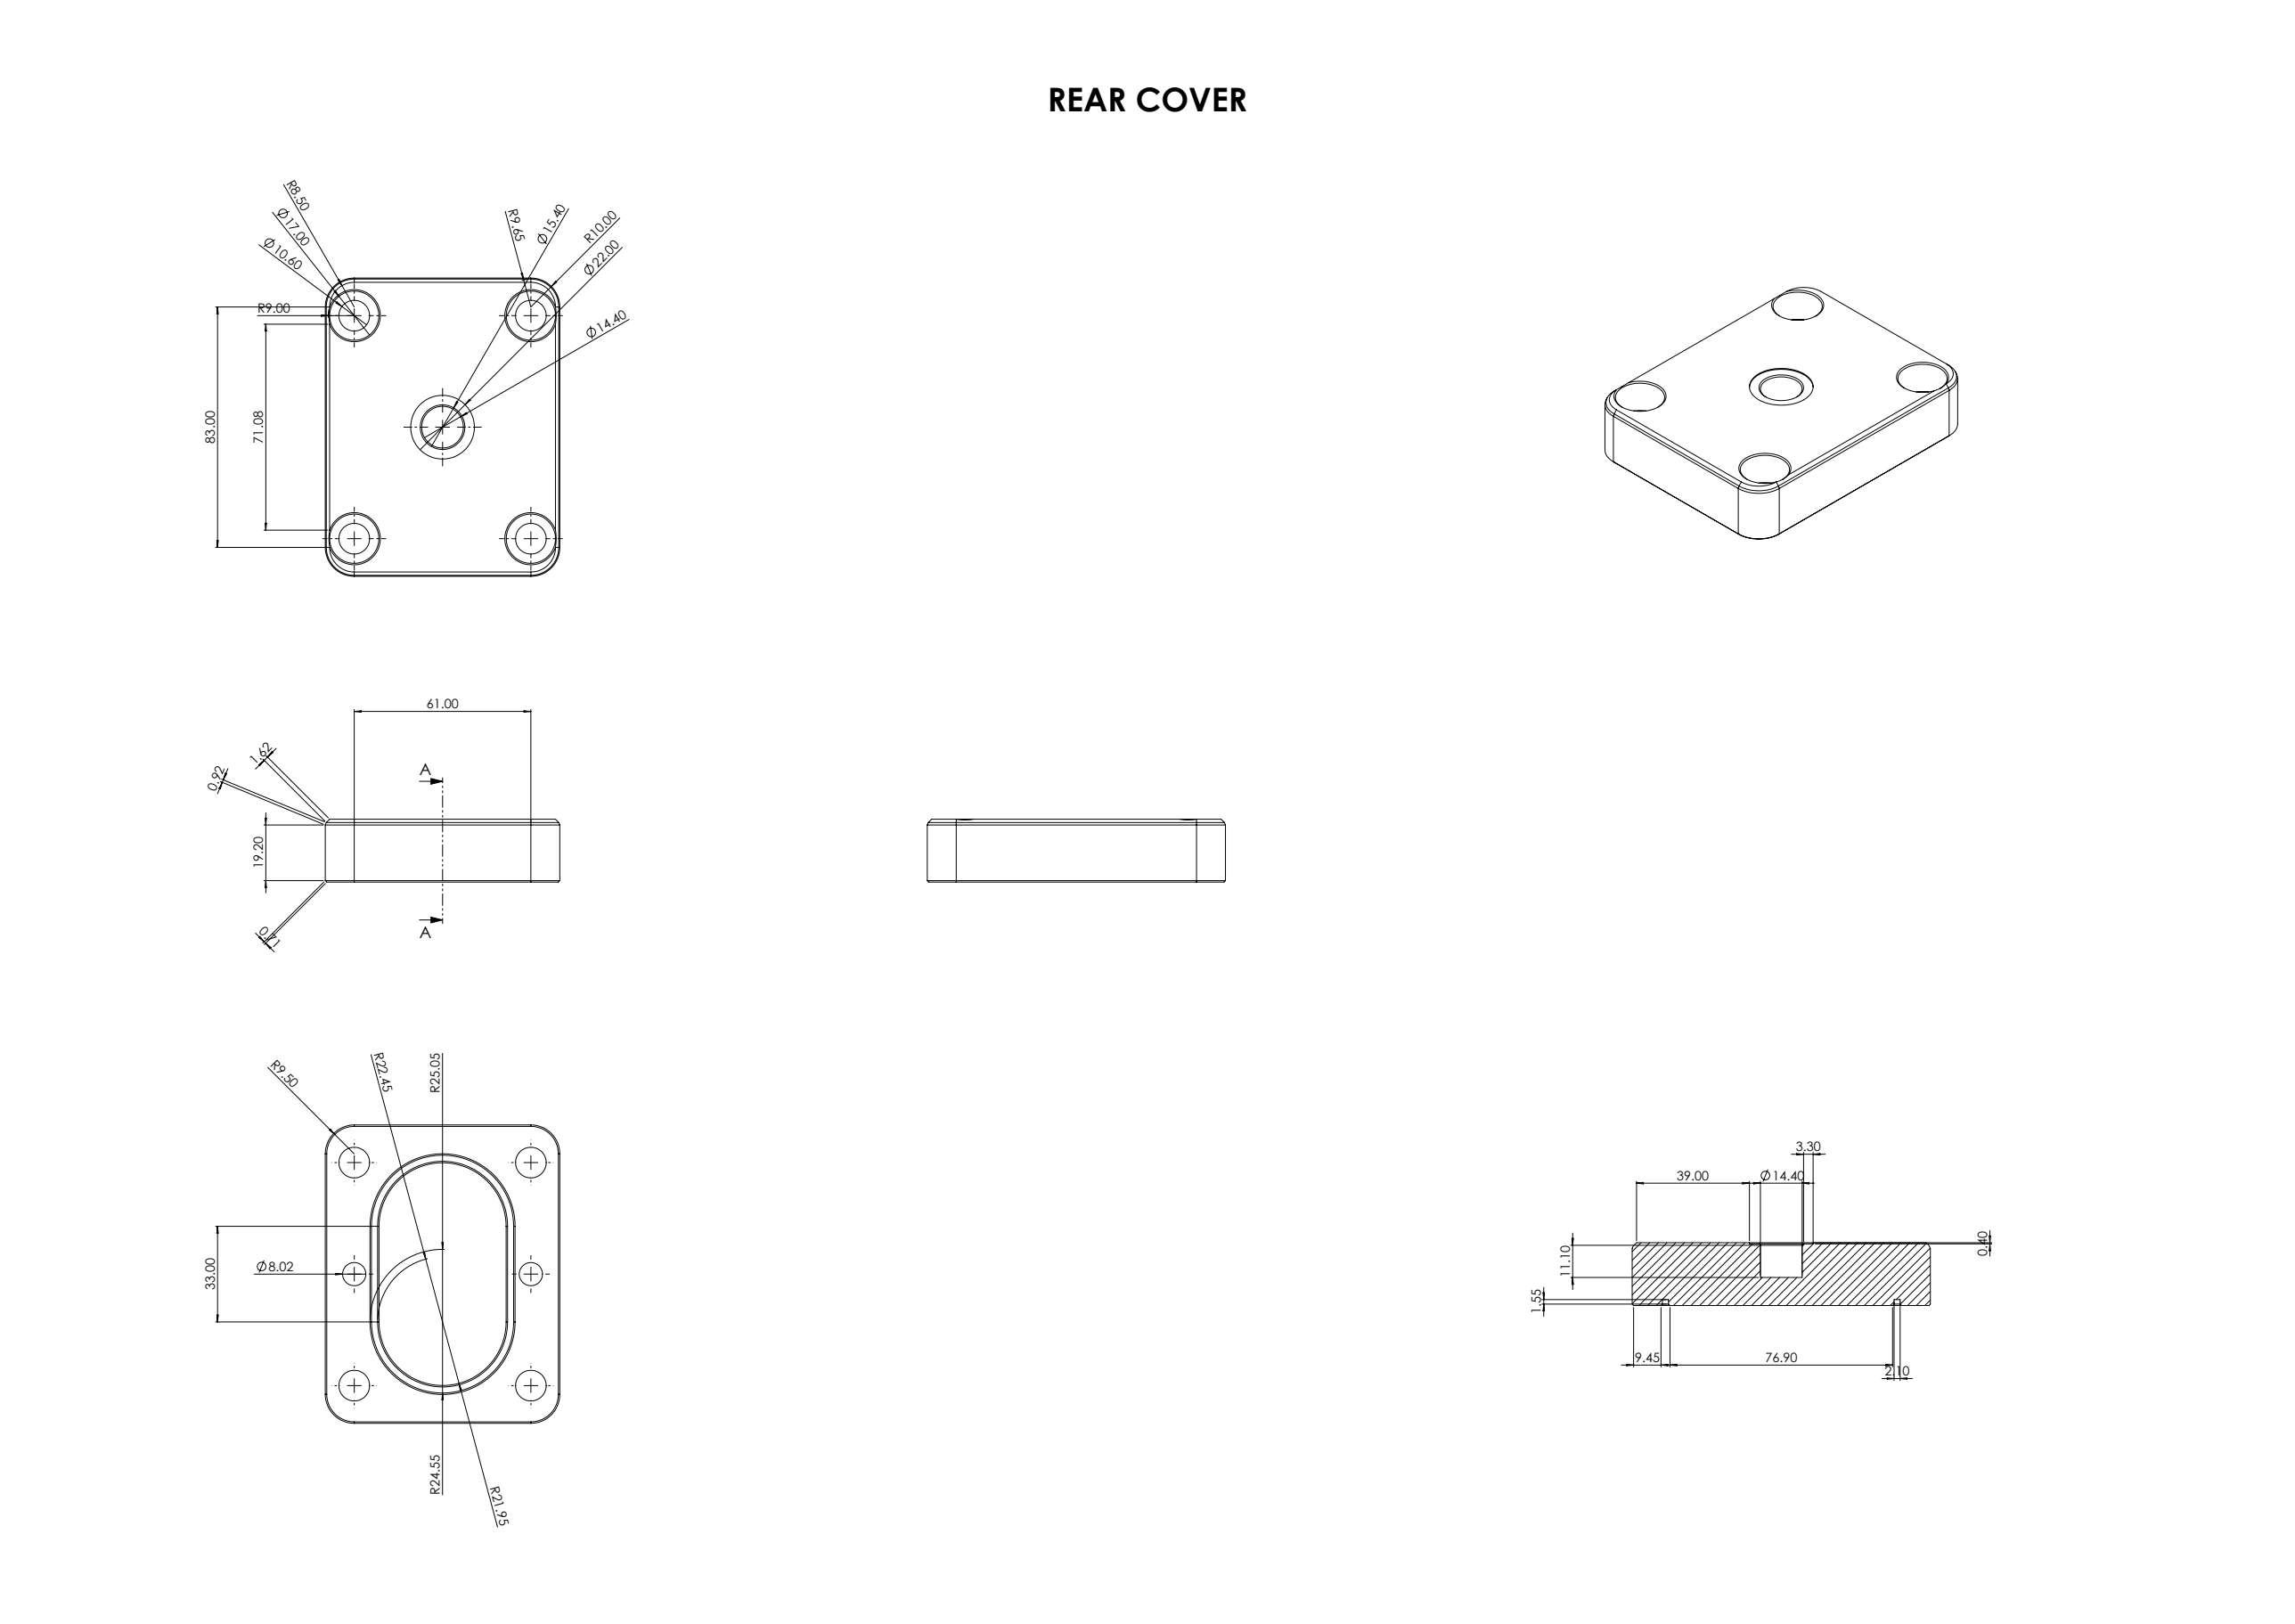
ISO-10303-21;
HEADER;
/* Generated by software containing ST-Developer
 * from STEP Tools, Inc. (www.steptools.com) 
 */

FILE_DESCRIPTION(
/* description */ (''),
/* implementation_level */ '2;1');

FILE_NAME(
/* name */ '03_Rear_Cover.step',
/* time_stamp */ '2026-10-26T06:59:52-07:00',
/* author */ (''),
/* organization */ (''),
/* preprocessor_version */ 'ST-DEVELOPER v20.2',
/* originating_system */ 'Autodesk Translation Framework v15.15.0.0',
/* authorisation */ '');

FILE_SCHEMA (('AUTOMOTIVE_DESIGN { 1 0 10303 214 3 1 1 }'));
ENDSEC;

DATA;
#10=MECHANICAL_DESIGN_GEOMETRIC_PRESENTATION_REPRESENTATION('',(#166),#46395);
#115=(
BOUNDED_CURVE()
B_SPLINE_CURVE(2,(#35773,#35774,#35775),.UNSPECIFIED.,.F.,.F.)
B_SPLINE_CURVE_WITH_KNOTS((3,3),(0.,0.297909382195316),.UNSPECIFIED.)
CURVE()
GEOMETRIC_REPRESENTATION_ITEM()
RATIONAL_B_SPLINE_CURVE((1.,1.,1.))
REPRESENTATION_ITEM('')
);
#116=(
BOUNDED_CURVE()
B_SPLINE_CURVE(2,(#35780,#35781,#35782),.UNSPECIFIED.,.F.,.F.)
B_SPLINE_CURVE_WITH_KNOTS((3,3),(0.297909382195316,0.595818764390632),
 .UNSPECIFIED.)
CURVE()
GEOMETRIC_REPRESENTATION_ITEM()
RATIONAL_B_SPLINE_CURVE((1.,1.,1.))
REPRESENTATION_ITEM('')
);
#117=(
BOUNDED_CURVE()
B_SPLINE_CURVE(2,(#35788,#35789,#35790),.UNSPECIFIED.,.F.,.F.)
B_SPLINE_CURVE_WITH_KNOTS((3,3),(0.297909382195316,0.595818764390632),
 .UNSPECIFIED.)
CURVE()
GEOMETRIC_REPRESENTATION_ITEM()
RATIONAL_B_SPLINE_CURVE((1.,1.,1.))
REPRESENTATION_ITEM('')
);
#118=(
BOUNDED_CURVE()
B_SPLINE_CURVE(2,(#35792,#35793,#35794),.UNSPECIFIED.,.F.,.F.)
B_SPLINE_CURVE_WITH_KNOTS((3,3),(0.,0.297909382195316),.UNSPECIFIED.)
CURVE()
GEOMETRIC_REPRESENTATION_ITEM()
RATIONAL_B_SPLINE_CURVE((1.,1.,1.))
REPRESENTATION_ITEM('')
);
#119=(
BOUNDED_CURVE()
B_SPLINE_CURVE(2,(#35820,#35821,#35822),.UNSPECIFIED.,.F.,.F.)
B_SPLINE_CURVE_WITH_KNOTS((3,3),(0.,0.297909382195316),.UNSPECIFIED.)
CURVE()
GEOMETRIC_REPRESENTATION_ITEM()
RATIONAL_B_SPLINE_CURVE((1.,1.,1.))
REPRESENTATION_ITEM('')
);
#120=(
BOUNDED_CURVE()
B_SPLINE_CURVE(2,(#35829,#35830,#35831),.UNSPECIFIED.,.F.,.F.)
B_SPLINE_CURVE_WITH_KNOTS((3,3),(0.297909382195316,0.595818764390632),
 .UNSPECIFIED.)
CURVE()
GEOMETRIC_REPRESENTATION_ITEM()
RATIONAL_B_SPLINE_CURVE((1.,1.,1.))
REPRESENTATION_ITEM('')
);
#121=(
BOUNDED_CURVE()
B_SPLINE_CURVE(2,(#35837,#35838,#35839),.UNSPECIFIED.,.F.,.F.)
B_SPLINE_CURVE_WITH_KNOTS((3,3),(0.297909382195316,0.595818764390632),
 .UNSPECIFIED.)
CURVE()
GEOMETRIC_REPRESENTATION_ITEM()
RATIONAL_B_SPLINE_CURVE((1.,1.,1.))
REPRESENTATION_ITEM('')
);
#122=(
BOUNDED_CURVE()
B_SPLINE_CURVE(2,(#35841,#35842,#35843),.UNSPECIFIED.,.F.,.F.)
B_SPLINE_CURVE_WITH_KNOTS((3,3),(0.,0.297909382195316),.UNSPECIFIED.)
CURVE()
GEOMETRIC_REPRESENTATION_ITEM()
RATIONAL_B_SPLINE_CURVE((1.,1.,1.))
REPRESENTATION_ITEM('')
);
#138=SHAPE_REPRESENTATION_RELATIONSHIP('SRR','None',#46458,#152);
#152=ADVANCED_BREP_SHAPE_REPRESENTATION('',(#180),#46383);
#166=STYLED_ITEM('',(#46610),#180);
#180=MANIFOLD_SOLID_BREP('Body1',#24939);
#494=CYLINDRICAL_SURFACE('',#25568,7.2);
#495=CYLINDRICAL_SURFACE('',#25578,24.55);
#496=CYLINDRICAL_SURFACE('',#25600,22.45);
#497=CYLINDRICAL_SURFACE('',#25608,8.5);
#498=CYLINDRICAL_SURFACE('',#25613,8.5);
#499=CYLINDRICAL_SURFACE('',#25620,8.5);
#500=CYLINDRICAL_SURFACE('',#25626,8.5);
#501=CYLINDRICAL_SURFACE('',#25641,9.99999999999999);
#502=CYLINDRICAL_SURFACE('',#25644,9.99999999999999);
#503=CYLINDRICAL_SURFACE('',#25672,22.45);
#504=CYLINDRICAL_SURFACE('',#25675,24.55);
#505=CYLINDRICAL_SURFACE('',#25679,11.);
#506=CYLINDRICAL_SURFACE('',#25681,4.01);
#507=CYLINDRICAL_SURFACE('',#25684,4.01);
#508=CYLINDRICAL_SURFACE('',#25687,5.3);
#509=CYLINDRICAL_SURFACE('',#25689,5.3);
#510=CYLINDRICAL_SURFACE('',#25691,5.3);
#511=CYLINDRICAL_SURFACE('',#25693,5.3);
#512=CYLINDRICAL_SURFACE('',#25699,9.99999999999999);
#513=CYLINDRICAL_SURFACE('',#25701,10.);
#631=FACE_BOUND('',#3353,.T.);
#632=FACE_BOUND('',#3362,.T.);
#633=FACE_BOUND('',#3363,.T.);
#634=FACE_BOUND('',#3364,.T.);
#635=FACE_BOUND('',#3365,.T.);
#636=FACE_BOUND('',#3366,.T.);
#637=FACE_BOUND('',#3367,.T.);
#638=FACE_BOUND('',#3368,.T.);
#639=FACE_BOUND('',#3413,.T.);
#640=FACE_BOUND('',#3419,.T.);
#641=FACE_BOUND('',#3431,.T.);
#642=FACE_BOUND('',#3433,.T.);
#643=FACE_BOUND('',#3435,.T.);
#644=FACE_BOUND('',#3437,.T.);
#778=PLANE('',#25566);
#779=PLANE('',#25570);
#780=PLANE('',#25574);
#781=PLANE('',#25580);
#782=PLANE('',#25581);
#783=PLANE('',#25592);
#784=PLANE('',#25596);
#785=PLANE('',#25602);
#786=PLANE('',#25603);
#787=PLANE('',#25607);
#788=PLANE('',#25619);
#789=PLANE('',#25630);
#790=PLANE('',#25633);
#791=PLANE('',#25636);
#792=PLANE('',#25639);
#793=PLANE('',#25640);
#794=PLANE('',#25643);
#795=PLANE('',#25646);
#796=PLANE('',#25649);
#797=PLANE('',#25652);
#798=PLANE('',#25656);
#799=PLANE('',#25662);
#800=PLANE('',#25667);
#801=PLANE('',#25670);
#802=PLANE('',#25674);
#803=PLANE('',#25677);
#804=PLANE('',#25678);
#805=PLANE('',#25680);
#806=PLANE('',#25683);
#807=PLANE('',#25686);
#808=PLANE('',#25695);
#809=PLANE('',#25696);
#810=PLANE('',#25697);
#811=PLANE('',#25698);
#812=PLANE('',#25700);
#813=PLANE('',#25702);
#1975=FACE_OUTER_BOUND('',#3351,.T.);
#1976=FACE_OUTER_BOUND('',#3352,.T.);
#1977=FACE_OUTER_BOUND('',#3354,.T.);
#1978=FACE_OUTER_BOUND('',#3355,.T.);
#1979=FACE_OUTER_BOUND('',#3356,.T.);
#1980=FACE_OUTER_BOUND('',#3357,.T.);
#1981=FACE_OUTER_BOUND('',#3358,.T.);
#1982=FACE_OUTER_BOUND('',#3359,.T.);
#1983=FACE_OUTER_BOUND('',#3360,.T.);
#1984=FACE_OUTER_BOUND('',#3361,.T.);
#1985=FACE_OUTER_BOUND('',#3369,.T.);
#1986=FACE_OUTER_BOUND('',#3370,.T.);
#1987=FACE_OUTER_BOUND('',#3371,.T.);
#1988=FACE_OUTER_BOUND('',#3372,.T.);
#1989=FACE_OUTER_BOUND('',#3373,.T.);
#1990=FACE_OUTER_BOUND('',#3374,.T.);
#1991=FACE_OUTER_BOUND('',#3375,.T.);
#1992=FACE_OUTER_BOUND('',#3376,.T.);
#1993=FACE_OUTER_BOUND('',#3377,.T.);
#1994=FACE_OUTER_BOUND('',#3378,.T.);
#1995=FACE_OUTER_BOUND('',#3379,.T.);
#1996=FACE_OUTER_BOUND('',#3380,.T.);
#1997=FACE_OUTER_BOUND('',#3381,.T.);
#1998=FACE_OUTER_BOUND('',#3382,.T.);
#1999=FACE_OUTER_BOUND('',#3383,.T.);
#2000=FACE_OUTER_BOUND('',#3384,.T.);
#2001=FACE_OUTER_BOUND('',#3385,.T.);
#2002=FACE_OUTER_BOUND('',#3386,.T.);
#2003=FACE_OUTER_BOUND('',#3387,.T.);
#2004=FACE_OUTER_BOUND('',#3388,.T.);
#2005=FACE_OUTER_BOUND('',#3389,.T.);
#2006=FACE_OUTER_BOUND('',#3390,.T.);
#2007=FACE_OUTER_BOUND('',#3391,.T.);
#2008=FACE_OUTER_BOUND('',#3392,.T.);
#2009=FACE_OUTER_BOUND('',#3393,.T.);
#2010=FACE_OUTER_BOUND('',#3394,.T.);
#2011=FACE_OUTER_BOUND('',#3395,.T.);
#2012=FACE_OUTER_BOUND('',#3396,.T.);
#2013=FACE_OUTER_BOUND('',#3397,.T.);
#2014=FACE_OUTER_BOUND('',#3398,.T.);
#2015=FACE_OUTER_BOUND('',#3399,.T.);
#2016=FACE_OUTER_BOUND('',#3400,.T.);
#2017=FACE_OUTER_BOUND('',#3401,.T.);
#2018=FACE_OUTER_BOUND('',#3402,.T.);
#2019=FACE_OUTER_BOUND('',#3403,.T.);
#2020=FACE_OUTER_BOUND('',#3404,.T.);
#2021=FACE_OUTER_BOUND('',#3405,.T.);
#2022=FACE_OUTER_BOUND('',#3406,.T.);
#2023=FACE_OUTER_BOUND('',#3407,.T.);
#2024=FACE_OUTER_BOUND('',#3408,.T.);
#2025=FACE_OUTER_BOUND('',#3409,.T.);
#2026=FACE_OUTER_BOUND('',#3410,.T.);
#2027=FACE_OUTER_BOUND('',#3411,.T.);
#2028=FACE_OUTER_BOUND('',#3412,.T.);
#2029=FACE_OUTER_BOUND('',#3414,.T.);
#2030=FACE_OUTER_BOUND('',#3415,.T.);
#2031=FACE_OUTER_BOUND('',#3416,.T.);
#2032=FACE_OUTER_BOUND('',#3417,.T.);
#2033=FACE_OUTER_BOUND('',#3418,.T.);
#2034=FACE_OUTER_BOUND('',#3420,.T.);
#2035=FACE_OUTER_BOUND('',#3421,.T.);
#2036=FACE_OUTER_BOUND('',#3422,.T.);
#2037=FACE_OUTER_BOUND('',#3423,.T.);
#2038=FACE_OUTER_BOUND('',#3424,.T.);
#2039=FACE_OUTER_BOUND('',#3425,.T.);
#2040=FACE_OUTER_BOUND('',#3426,.T.);
#2041=FACE_OUTER_BOUND('',#3427,.T.);
#2042=FACE_OUTER_BOUND('',#3428,.T.);
#2043=FACE_OUTER_BOUND('',#3429,.T.);
#2044=FACE_OUTER_BOUND('',#3430,.T.);
#2045=FACE_OUTER_BOUND('',#3432,.T.);
#2046=FACE_OUTER_BOUND('',#3434,.T.);
#2047=FACE_OUTER_BOUND('',#3436,.T.);
#2048=FACE_OUTER_BOUND('',#3438,.T.);
#2049=FACE_OUTER_BOUND('',#3439,.T.);
#2050=FACE_OUTER_BOUND('',#3440,.T.);
#2051=FACE_OUTER_BOUND('',#3441,.T.);
#3351=EDGE_LOOP('',(#17582,#17583,#17584,#17585));
#3352=EDGE_LOOP('',(#17586));
#3353=EDGE_LOOP('',(#17587));
#3354=EDGE_LOOP('',(#17588,#17589,#17590,#17591));
#3355=EDGE_LOOP('',(#17592,#17593,#17594,#17595));
#3356=EDGE_LOOP('',(#17596,#17597,#17598,#17599));
#3357=EDGE_LOOP('',(#17600,#17601,#17602,#17603));
#3358=EDGE_LOOP('',(#17604,#17605,#17606,#17607));
#3359=EDGE_LOOP('',(#17608,#17609,#17610,#17611));
#3360=EDGE_LOOP('',(#17612,#17613,#17614,#17615));
#3361=EDGE_LOOP('',(#17616,#17617,#17618,#17619,#17620,#17621,#17622,#17623));
#3362=EDGE_LOOP('',(#17624));
#3363=EDGE_LOOP('',(#17625));
#3364=EDGE_LOOP('',(#17626));
#3365=EDGE_LOOP('',(#17627));
#3366=EDGE_LOOP('',(#17628));
#3367=EDGE_LOOP('',(#17629));
#3368=EDGE_LOOP('',(#17630,#17631,#17632,#17633));
#3369=EDGE_LOOP('',(#17634,#17635,#17636,#17637));
#3370=EDGE_LOOP('',(#17638,#17639,#17640,#17641));
#3371=EDGE_LOOP('',(#17642,#17643,#17644,#17645));
#3372=EDGE_LOOP('',(#17646,#17647,#17648,#17649));
#3373=EDGE_LOOP('',(#17650,#17651,#17652,#17653));
#3374=EDGE_LOOP('',(#17654,#17655,#17656,#17657));
#3375=EDGE_LOOP('',(#17658,#17659,#17660,#17661));
#3376=EDGE_LOOP('',(#17662,#17663,#17664,#17665,#17666,#17667));
#3377=EDGE_LOOP('',(#17668,#17669,#17670,#17671,#17672,#17673,#17674,#17675,
#17676,#17677));
#3378=EDGE_LOOP('',(#17678,#17679,#17680,#17681));
#3379=EDGE_LOOP('',(#17682,#17683,#17684,#17685,#17686,#17687));
#3380=EDGE_LOOP('',(#17688,#17689,#17690,#17691));
#3381=EDGE_LOOP('',(#17692,#17693,#17694,#17695,#17696,#17697,#17698));
#3382=EDGE_LOOP('',(#17699,#17700,#17701,#17702,#17703,#17704,#17705,#17706,
#17707,#17708));
#3383=EDGE_LOOP('',(#17709,#17710,#17711,#17712,#17713));
#3384=EDGE_LOOP('',(#17714,#17715,#17716,#17717,#17718,#17719,#17720));
#3385=EDGE_LOOP('',(#17721,#17722,#17723,#17724,#17725));
#3386=EDGE_LOOP('',(#17726,#17727,#17728,#17729));
#3387=EDGE_LOOP('',(#17730,#17731,#17732,#17733));
#3388=EDGE_LOOP('',(#17734,#17735,#17736,#17737));
#3389=EDGE_LOOP('',(#17738,#17739,#17740,#17741));
#3390=EDGE_LOOP('',(#17742,#17743,#17744,#17745));
#3391=EDGE_LOOP('',(#17746,#17747,#17748,#17749));
#3392=EDGE_LOOP('',(#17750,#17751,#17752,#17753));
#3393=EDGE_LOOP('',(#17754,#17755,#17756,#17757));
#3394=EDGE_LOOP('',(#17758,#17759,#17760,#17761));
#3395=EDGE_LOOP('',(#17762,#17763,#17764,#17765));
#3396=EDGE_LOOP('',(#17766,#17767,#17768,#17769));
#3397=EDGE_LOOP('',(#17770,#17771,#17772,#17773));
#3398=EDGE_LOOP('',(#17774,#17775,#17776,#17777));
#3399=EDGE_LOOP('',(#17778,#17779,#17780,#17781));
#3400=EDGE_LOOP('',(#17782,#17783,#17784,#17785));
#3401=EDGE_LOOP('',(#17786,#17787,#17788,#17789));
#3402=EDGE_LOOP('',(#17790,#17791,#17792,#17793));
#3403=EDGE_LOOP('',(#17794,#17795,#17796,#17797));
#3404=EDGE_LOOP('',(#17798,#17799,#17800,#17801));
#3405=EDGE_LOOP('',(#17802,#17803,#17804,#17805));
#3406=EDGE_LOOP('',(#17806,#17807,#17808,#17809));
#3407=EDGE_LOOP('',(#17810,#17811,#17812,#17813));
#3408=EDGE_LOOP('',(#17814,#17815,#17816,#17817));
#3409=EDGE_LOOP('',(#17818,#17819,#17820,#17821));
#3410=EDGE_LOOP('',(#17822,#17823,#17824,#17825));
#3411=EDGE_LOOP('',(#17826,#17827,#17828,#17829));
#3412=EDGE_LOOP('',(#17830,#17831,#17832,#17833,#17834,#17835,#17836,#17837,
#17838,#17839,#17840,#17841,#17842,#17843,#17844,#17845));
#3413=EDGE_LOOP('',(#17846));
#3414=EDGE_LOOP('',(#17847,#17848,#17849,#17850));
#3415=EDGE_LOOP('',(#17851,#17852,#17853,#17854));
#3416=EDGE_LOOP('',(#17855,#17856,#17857,#17858));
#3417=EDGE_LOOP('',(#17859,#17860,#17861,#17862));
#3418=EDGE_LOOP('',(#17863,#17864,#17865,#17866));
#3419=EDGE_LOOP('',(#17867,#17868,#17869,#17870));
#3420=EDGE_LOOP('',(#17871,#17872,#17873,#17874));
#3421=EDGE_LOOP('',(#17875));
#3422=EDGE_LOOP('',(#17876,#17877,#17878,#17879));
#3423=EDGE_LOOP('',(#17880));
#3424=EDGE_LOOP('',(#17881,#17882,#17883,#17884));
#3425=EDGE_LOOP('',(#17885));
#3426=EDGE_LOOP('',(#17886,#17887,#17888,#17889));
#3427=EDGE_LOOP('',(#17890,#17891,#17892,#17893));
#3428=EDGE_LOOP('',(#17894,#17895,#17896,#17897));
#3429=EDGE_LOOP('',(#17898,#17899,#17900,#17901));
#3430=EDGE_LOOP('',(#17902));
#3431=EDGE_LOOP('',(#17903));
#3432=EDGE_LOOP('',(#17904));
#3433=EDGE_LOOP('',(#17905));
#3434=EDGE_LOOP('',(#17906));
#3435=EDGE_LOOP('',(#17907));
#3436=EDGE_LOOP('',(#17908));
#3437=EDGE_LOOP('',(#17909));
#3438=EDGE_LOOP('',(#17910,#17911,#17912,#17913));
#3439=EDGE_LOOP('',(#17914,#17915,#17916,#17917));
#3440=EDGE_LOOP('',(#17918,#17919,#17920,#17921));
#3441=EDGE_LOOP('',(#17922,#17923,#17924,#17925));
#4766=LINE('',#35663,#7635);
#4767=LINE('',#35670,#7636);
#4768=LINE('',#35675,#7637);
#4769=LINE('',#35677,#7638);
#4770=LINE('',#35679,#7639);
#4771=LINE('',#35680,#7640);
#4772=LINE('',#35684,#7641);
#4773=LINE('',#35690,#7642);
#4774=LINE('',#35691,#7643);
#4775=LINE('',#35692,#7644);
#4776=LINE('',#35698,#7645);
#4777=LINE('',#35701,#7646);
#4778=LINE('',#35704,#7647);
#4779=LINE('',#35705,#7648);
#4780=LINE('',#35711,#7649);
#4781=LINE('',#35715,#7650);
#4782=LINE('',#35719,#7651);
#4783=LINE('',#35722,#7652);
#4784=LINE('',#35738,#7653);
#4785=LINE('',#35740,#7654);
#4786=LINE('',#35742,#7655);
#4787=LINE('',#35743,#7656);
#4788=LINE('',#35747,#7657);
#4789=LINE('',#35753,#7658);
#4790=LINE('',#35754,#7659);
#4791=LINE('',#35755,#7660);
#4792=LINE('',#35761,#7661);
#4793=LINE('',#35764,#7662);
#4794=LINE('',#35767,#7663);
#4795=LINE('',#35768,#7664);
#4796=LINE('',#35777,#7665);
#4797=LINE('',#35786,#7666);
#4798=LINE('',#35796,#7667);
#4799=LINE('',#35798,#7668);
#4800=LINE('',#35800,#7669);
#4801=LINE('',#35802,#7670);
#4802=LINE('',#35803,#7671);
#4803=LINE('',#35806,#7672);
#4804=LINE('',#35810,#7673);
#4805=LINE('',#35815,#7674);
#4806=LINE('',#35824,#7675);
#4807=LINE('',#35835,#7676);
#4808=LINE('',#35845,#7677);
#4809=LINE('',#35847,#7678);
#4810=LINE('',#35849,#7679);
#4811=LINE('',#35851,#7680);
#4812=LINE('',#35852,#7681);
#4813=LINE('',#35855,#7682);
#4814=LINE('',#35859,#7683);
#4815=LINE('',#35866,#7684);
#4816=LINE('',#35870,#7685);
#4817=LINE('',#35873,#7686);
#4818=LINE('',#35876,#7687);
#4819=LINE('',#35877,#7688);
#4820=LINE('',#35880,#7689);
#4821=LINE('',#35884,#7690);
#4822=LINE('',#35885,#7691);
#4823=LINE('',#35888,#7692);
#4824=LINE('',#35892,#7693);
#4825=LINE('',#35893,#7694);
#4826=LINE('',#35896,#7695);
#4827=LINE('',#35899,#7696);
#4828=LINE('',#35902,#7697);
#4829=LINE('',#35904,#7698);
#4830=LINE('',#35905,#7699);
#4831=LINE('',#35908,#7700);
#4832=LINE('',#35912,#7701);
#4833=LINE('',#35913,#7702);
#4834=LINE('',#35916,#7703);
#4835=LINE('',#35919,#7704);
#4836=LINE('',#35920,#7705);
#4837=LINE('',#35923,#7706);
#4838=LINE('',#35927,#7707);
#4839=LINE('',#35928,#7708);
#4840=LINE('',#35930,#7709);
#4841=LINE('',#35934,#7710);
#4842=LINE('',#35935,#7711);
#4843=LINE('',#35939,#7712);
#4844=LINE('',#35945,#7713);
#4845=LINE('',#35946,#7714);
#4846=LINE('',#35947,#7715);
#4847=LINE('',#35953,#7716);
#4848=LINE('',#35957,#7717);
#4849=LINE('',#35958,#7718);
#4850=LINE('',#35963,#7719);
#4851=LINE('',#35967,#7720);
#4852=LINE('',#35968,#7721);
#4853=LINE('',#35976,#7722);
#4854=LINE('',#35979,#7723);
#4855=LINE('',#35982,#7724);
#4856=LINE('',#35985,#7725);
#4857=LINE('',#35988,#7726);
#4858=LINE('',#35992,#7727);
#4859=LINE('',#35997,#7728);
#4860=LINE('',#36003,#7729);
#4861=LINE('',#36007,#7730);
#4862=LINE('',#36011,#7731);
#4863=LINE('',#36015,#7732);
#4864=LINE('',#36021,#7733);
#4865=LINE('',#36023,#7734);
#4866=LINE('',#36025,#7735);
#7635=VECTOR('',#28083,7.45);
#7636=VECTOR('',#28092,7.2);
#7637=VECTOR('',#28097,10.);
#7638=VECTOR('',#28098,10.);
#7639=VECTOR('',#28099,10.);
#7640=VECTOR('',#28100,10.);
#7641=VECTOR('',#28103,10.);
#7642=VECTOR('',#28110,10.);
#7643=VECTOR('',#28111,10.);
#7644=VECTOR('',#28112,10.);
#7645=VECTOR('',#28121,10.);
#7646=VECTOR('',#28124,10.);
#7647=VECTOR('',#28127,10.);
#7648=VECTOR('',#28128,10.);
#7649=VECTOR('',#28133,10.);
#7650=VECTOR('',#28136,10.);
#7651=VECTOR('',#28139,10.);
#7652=VECTOR('',#28142,10.);
#7653=VECTOR('',#28157,10.);
#7654=VECTOR('',#28158,10.);
#7655=VECTOR('',#28159,10.);
#7656=VECTOR('',#28160,10.);
#7657=VECTOR('',#28163,10.);
#7658=VECTOR('',#28170,10.);
#7659=VECTOR('',#28171,10.);
#7660=VECTOR('',#28172,10.);
#7661=VECTOR('',#28181,10.);
#7662=VECTOR('',#28184,10.);
#7663=VECTOR('',#28187,10.);
#7664=VECTOR('',#28188,10.);
#7665=VECTOR('',#28193,8.75);
#7666=VECTOR('',#28200,10.);
#7667=VECTOR('',#28201,10.);
#7668=VECTOR('',#28202,10.);
#7669=VECTOR('',#28203,10.);
#7670=VECTOR('',#28204,10.);
#7671=VECTOR('',#28205,10.);
#7672=VECTOR('',#28208,8.5);
#7673=VECTOR('',#28213,8.75);
#7674=VECTOR('',#28220,8.5);
#7675=VECTOR('',#28225,8.75);
#7676=VECTOR('',#28234,10.);
#7677=VECTOR('',#28235,10.);
#7678=VECTOR('',#28236,10.);
#7679=VECTOR('',#28237,10.);
#7680=VECTOR('',#28238,10.);
#7681=VECTOR('',#28239,10.);
#7682=VECTOR('',#28242,8.5);
#7683=VECTOR('',#28247,8.75);
#7684=VECTOR('',#28256,8.5);
#7685=VECTOR('',#28261,10.);
#7686=VECTOR('',#28264,10.);
#7687=VECTOR('',#28267,10.);
#7688=VECTOR('',#28268,10.);
#7689=VECTOR('',#28271,10.);
#7690=VECTOR('',#28276,10.);
#7691=VECTOR('',#28277,10.);
#7692=VECTOR('',#28280,10.);
#7693=VECTOR('',#28285,10.);
#7694=VECTOR('',#28286,10.);
#7695=VECTOR('',#28289,10.);
#7696=VECTOR('',#28294,10.);
#7697=VECTOR('',#28297,10.);
#7698=VECTOR('',#28298,10.);
#7699=VECTOR('',#28299,10.);
#7700=VECTOR('',#28302,10.);
#7701=VECTOR('',#28307,10.);
#7702=VECTOR('',#28308,10.);
#7703=VECTOR('',#28311,10.);
#7704=VECTOR('',#28316,10.);
#7705=VECTOR('',#28317,10.);
#7706=VECTOR('',#28320,10.);
#7707=VECTOR('',#28325,10.);
#7708=VECTOR('',#28326,10.);
#7709=VECTOR('',#28329,10.);
#7710=VECTOR('',#28334,10.);
#7711=VECTOR('',#28335,10.);
#7712=VECTOR('',#28338,10.);
#7713=VECTOR('',#28345,10.);
#7714=VECTOR('',#28346,10.);
#7715=VECTOR('',#28347,10.);
#7716=VECTOR('',#28356,10.);
#7717=VECTOR('',#28361,10.);
#7718=VECTOR('',#28362,10.);
#7719=VECTOR('',#28369,10.);
#7720=VECTOR('',#28374,10.);
#7721=VECTOR('',#28375,10.);
#7722=VECTOR('',#28386,10.);
#7723=VECTOR('',#28391,10.);
#7724=VECTOR('',#28394,10.);
#7725=VECTOR('',#28399,10.);
#7726=VECTOR('',#28404,11.);
#7727=VECTOR('',#28409,4.01);
#7728=VECTOR('',#28416,4.01);
#7729=VECTOR('',#28425,5.3);
#7730=VECTOR('',#28430,5.3);
#7731=VECTOR('',#28435,5.3);
#7732=VECTOR('',#28440,5.3);
#7733=VECTOR('',#28451,10.);
#7734=VECTOR('',#28454,10.);
#7735=VECTOR('',#28457,10.);
#10505=CIRCLE('',#25564,7.2);
#10506=CIRCLE('',#25565,7.7);
#10507=CIRCLE('',#25567,11.);
#10508=CIRCLE('',#25569,7.2);
#10509=CIRCLE('',#25572,25.05);
#10510=CIRCLE('',#25573,24.55);
#10511=CIRCLE('',#25576,25.05);
#10512=CIRCLE('',#25577,24.55);
#10513=CIRCLE('',#25579,24.55);
#10514=CIRCLE('',#25582,9.49999999999999);
#10515=CIRCLE('',#25583,9.49999999999999);
#10516=CIRCLE('',#25584,9.49999999999999);
#10517=CIRCLE('',#25585,9.5);
#10518=CIRCLE('',#25586,5.3);
#10519=CIRCLE('',#25587,5.3);
#10520=CIRCLE('',#25588,5.3);
#10521=CIRCLE('',#25589,5.3);
#10522=CIRCLE('',#25590,4.01);
#10523=CIRCLE('',#25591,4.01);
#10524=CIRCLE('',#25594,21.95);
#10525=CIRCLE('',#25595,22.45);
#10526=CIRCLE('',#25598,21.95);
#10527=CIRCLE('',#25599,22.45);
#10528=CIRCLE('',#25601,22.45);
#10529=CIRCLE('',#25605,8.5);
#10530=CIRCLE('',#25606,9.);
#10531=CIRCLE('',#25609,8.5);
#10532=CIRCLE('',#25611,8.5);
#10533=CIRCLE('',#25612,9.);
#10534=CIRCLE('',#25614,8.5);
#10535=CIRCLE('',#25616,8.5);
#10536=CIRCLE('',#25617,8.5);
#10537=CIRCLE('',#25618,9.);
#10538=CIRCLE('',#25621,8.5);
#10539=CIRCLE('',#25623,8.5);
#10540=CIRCLE('',#25624,8.5);
#10541=CIRCLE('',#25625,9.);
#10542=CIRCLE('',#25627,8.5);
#10543=CIRCLE('',#25629,9.99999999999999);
#10544=CIRCLE('',#25632,10.);
#10545=CIRCLE('',#25635,9.99999999999999);
#10546=CIRCLE('',#25638,9.99999999999999);
#10547=CIRCLE('',#25642,9.99999999999999);
#10548=CIRCLE('',#25645,9.99999999999999);
#10549=CIRCLE('',#25648,9.64644660940673);
#10550=CIRCLE('',#25651,9.64644660940672);
#10551=CIRCLE('',#25654,9.64644660940673);
#10552=CIRCLE('',#25655,10.);
#10553=CIRCLE('',#25658,9.64644660940671);
#10554=CIRCLE('',#25659,9.99999999999999);
#10555=CIRCLE('',#25661,8.49999999999999);
#10556=CIRCLE('',#25664,8.49999999999999);
#10557=CIRCLE('',#25666,8.49999999999999);
#10558=CIRCLE('',#25669,8.49999999999999);
#10559=CIRCLE('',#25671,11.);
#10560=CIRCLE('',#25673,22.45);
#10561=CIRCLE('',#25676,24.55);
#10562=CIRCLE('',#25682,4.01);
#10563=CIRCLE('',#25685,4.01);
#10564=CIRCLE('',#25688,5.3);
#10565=CIRCLE('',#25690,5.3);
#10566=CIRCLE('',#25692,5.3);
#10567=CIRCLE('',#25694,5.3);
#11054=VERTEX_POINT('',#35660);
#11055=VERTEX_POINT('',#35662);
#11056=VERTEX_POINT('',#35666);
#11057=VERTEX_POINT('',#35669);
#11058=VERTEX_POINT('',#35673);
#11059=VERTEX_POINT('',#35674);
#11060=VERTEX_POINT('',#35676);
#11061=VERTEX_POINT('',#35678);
#11062=VERTEX_POINT('',#35682);
#11063=VERTEX_POINT('',#35683);
#11064=VERTEX_POINT('',#35688);
#11065=VERTEX_POINT('',#35689);
#11066=VERTEX_POINT('',#35697);
#11067=VERTEX_POINT('',#35699);
#11068=VERTEX_POINT('',#35703);
#11069=VERTEX_POINT('',#35707);
#11070=VERTEX_POINT('',#35708);
#11071=VERTEX_POINT('',#35710);
#11072=VERTEX_POINT('',#35712);
#11073=VERTEX_POINT('',#35714);
#11074=VERTEX_POINT('',#35716);
#11075=VERTEX_POINT('',#35718);
#11076=VERTEX_POINT('',#35720);
#11077=VERTEX_POINT('',#35723);
#11078=VERTEX_POINT('',#35725);
#11079=VERTEX_POINT('',#35727);
#11080=VERTEX_POINT('',#35729);
#11081=VERTEX_POINT('',#35731);
#11082=VERTEX_POINT('',#35733);
#11083=VERTEX_POINT('',#35736);
#11084=VERTEX_POINT('',#35737);
#11085=VERTEX_POINT('',#35739);
#11086=VERTEX_POINT('',#35741);
#11087=VERTEX_POINT('',#35745);
#11088=VERTEX_POINT('',#35746);
#11089=VERTEX_POINT('',#35751);
#11090=VERTEX_POINT('',#35752);
#11091=VERTEX_POINT('',#35760);
#11092=VERTEX_POINT('',#35762);
#11093=VERTEX_POINT('',#35766);
#11094=VERTEX_POINT('',#35771);
#11095=VERTEX_POINT('',#35772);
#11096=VERTEX_POINT('',#35776);
#11097=VERTEX_POINT('',#35779);
#11098=VERTEX_POINT('',#35785);
#11099=VERTEX_POINT('',#35787);
#11100=VERTEX_POINT('',#35791);
#11101=VERTEX_POINT('',#35795);
#11102=VERTEX_POINT('',#35797);
#11103=VERTEX_POINT('',#35799);
#11104=VERTEX_POINT('',#35801);
#11105=VERTEX_POINT('',#35805);
#11106=VERTEX_POINT('',#35809);
#11107=VERTEX_POINT('',#35814);
#11108=VERTEX_POINT('',#35818);
#11109=VERTEX_POINT('',#35819);
#11110=VERTEX_POINT('',#35823);
#11111=VERTEX_POINT('',#35825);
#11112=VERTEX_POINT('',#35828);
#11113=VERTEX_POINT('',#35834);
#11114=VERTEX_POINT('',#35836);
#11115=VERTEX_POINT('',#35840);
#11116=VERTEX_POINT('',#35844);
#11117=VERTEX_POINT('',#35846);
#11118=VERTEX_POINT('',#35848);
#11119=VERTEX_POINT('',#35850);
#11120=VERTEX_POINT('',#35854);
#11121=VERTEX_POINT('',#35858);
#11122=VERTEX_POINT('',#35860);
#11123=VERTEX_POINT('',#35865);
#11124=VERTEX_POINT('',#35869);
#11125=VERTEX_POINT('',#35871);
#11126=VERTEX_POINT('',#35875);
#11127=VERTEX_POINT('',#35879);
#11128=VERTEX_POINT('',#35883);
#11129=VERTEX_POINT('',#35887);
#11130=VERTEX_POINT('',#35891);
#11131=VERTEX_POINT('',#35895);
#11132=VERTEX_POINT('',#35901);
#11133=VERTEX_POINT('',#35903);
#11134=VERTEX_POINT('',#35907);
#11135=VERTEX_POINT('',#35911);
#11136=VERTEX_POINT('',#35915);
#11137=VERTEX_POINT('',#35922);
#11138=VERTEX_POINT('',#35926);
#11139=VERTEX_POINT('',#35933);
#11140=VERTEX_POINT('',#35937);
#11141=VERTEX_POINT('',#35938);
#11142=VERTEX_POINT('',#35943);
#11143=VERTEX_POINT('',#35944);
#11144=VERTEX_POINT('',#35952);
#11145=VERTEX_POINT('',#35956);
#11146=VERTEX_POINT('',#35962);
#11147=VERTEX_POINT('',#35966);
#11148=VERTEX_POINT('',#35972);
#11149=VERTEX_POINT('',#35975);
#11150=VERTEX_POINT('',#35981);
#11151=VERTEX_POINT('',#35991);
#11152=VERTEX_POINT('',#35996);
#11153=VERTEX_POINT('',#36001);
#11154=VERTEX_POINT('',#36005);
#11155=VERTEX_POINT('',#36009);
#11156=VERTEX_POINT('',#36013);
#13544=EDGE_CURVE('',#11054,#11054,#10505,.T.);
#13545=EDGE_CURVE('',#11054,#11055,#4766,.T.);
#13546=EDGE_CURVE('',#11055,#11055,#10506,.T.);
#13547=EDGE_CURVE('',#11056,#11056,#10507,.T.);
#13548=EDGE_CURVE('',#11054,#11057,#4767,.T.);
#13549=EDGE_CURVE('',#11057,#11057,#10508,.T.);
#13550=EDGE_CURVE('',#11058,#11059,#4768,.T.);
#13551=EDGE_CURVE('',#11059,#11060,#4769,.T.);
#13552=EDGE_CURVE('',#11060,#11061,#4770,.T.);
#13553=EDGE_CURVE('',#11061,#11058,#4771,.T.);
#13554=EDGE_CURVE('',#11062,#11063,#4772,.T.);
#13555=EDGE_CURVE('',#11063,#11059,#10509,.T.);
#13556=EDGE_CURVE('',#11058,#11062,#10510,.T.);
#13557=EDGE_CURVE('',#11064,#11065,#4773,.T.);
#13558=EDGE_CURVE('',#11065,#11063,#4774,.T.);
#13559=EDGE_CURVE('',#11062,#11064,#4775,.T.);
#13560=EDGE_CURVE('',#11060,#11065,#10511,.T.);
#13561=EDGE_CURVE('',#11064,#11061,#10512,.T.);
#13562=EDGE_CURVE('',#11058,#11066,#4776,.T.);
#13563=EDGE_CURVE('',#11066,#11067,#10513,.T.);
#13564=EDGE_CURVE('',#11062,#11067,#4777,.T.);
#13565=EDGE_CURVE('',#11061,#11068,#4778,.T.);
#13566=EDGE_CURVE('',#11068,#11066,#4779,.T.);
#13567=EDGE_CURVE('',#11069,#11070,#10514,.T.);
#13568=EDGE_CURVE('',#11071,#11069,#4780,.T.);
#13569=EDGE_CURVE('',#11072,#11071,#10515,.T.);
#13570=EDGE_CURVE('',#11073,#11072,#4781,.T.);
#13571=EDGE_CURVE('',#11074,#11073,#10516,.T.);
#13572=EDGE_CURVE('',#11075,#11074,#4782,.T.);
#13573=EDGE_CURVE('',#11076,#11075,#10517,.T.);
#13574=EDGE_CURVE('',#11070,#11076,#4783,.T.);
#13575=EDGE_CURVE('',#11077,#11077,#10518,.T.);
#13576=EDGE_CURVE('',#11078,#11078,#10519,.T.);
#13577=EDGE_CURVE('',#11079,#11079,#10520,.T.);
#13578=EDGE_CURVE('',#11080,#11080,#10521,.T.);
#13579=EDGE_CURVE('',#11081,#11081,#10522,.T.);
#13580=EDGE_CURVE('',#11082,#11082,#10523,.T.);
#13581=EDGE_CURVE('',#11083,#11084,#4784,.T.);
#13582=EDGE_CURVE('',#11084,#11085,#4785,.T.);
#13583=EDGE_CURVE('',#11085,#11086,#4786,.T.);
#13584=EDGE_CURVE('',#11086,#11083,#4787,.T.);
#13585=EDGE_CURVE('',#11087,#11088,#4788,.T.);
#13586=EDGE_CURVE('',#11088,#11084,#10524,.T.);
#13587=EDGE_CURVE('',#11083,#11087,#10525,.T.);
#13588=EDGE_CURVE('',#11089,#11090,#4789,.T.);
#13589=EDGE_CURVE('',#11090,#11088,#4790,.T.);
#13590=EDGE_CURVE('',#11087,#11089,#4791,.T.);
#13591=EDGE_CURVE('',#11085,#11090,#10526,.T.);
#13592=EDGE_CURVE('',#11089,#11086,#10527,.T.);
#13593=EDGE_CURVE('',#11083,#11091,#4792,.T.);
#13594=EDGE_CURVE('',#11091,#11092,#10528,.T.);
#13595=EDGE_CURVE('',#11087,#11092,#4793,.T.);
#13596=EDGE_CURVE('',#11086,#11093,#4794,.T.);
#13597=EDGE_CURVE('',#11093,#11091,#4795,.T.);
#13598=EDGE_CURVE('',#11094,#11095,#115,.T.);
#13599=EDGE_CURVE('',#11095,#11096,#4796,.T.);
#13600=EDGE_CURVE('',#11096,#11096,#10529,.T.);
#13601=EDGE_CURVE('',#11095,#11097,#116,.T.);
#13602=EDGE_CURVE('',#11097,#11094,#10530,.T.);
#13603=EDGE_CURVE('',#11094,#11098,#4797,.T.);
#13604=EDGE_CURVE('',#11099,#11098,#117,.T.);
#13605=EDGE_CURVE('',#11100,#11099,#118,.T.);
#13606=EDGE_CURVE('',#11100,#11101,#4798,.T.);
#13607=EDGE_CURVE('',#11102,#11101,#4799,.T.);
#13608=EDGE_CURVE('',#11103,#11102,#4800,.T.);
#13609=EDGE_CURVE('',#11103,#11104,#4801,.T.);
#13610=EDGE_CURVE('',#11104,#11097,#4802,.T.);
#13611=EDGE_CURVE('',#11096,#11105,#4803,.T.);
#13612=EDGE_CURVE('',#11105,#11105,#10531,.T.);
#13613=EDGE_CURVE('',#11099,#11106,#4804,.T.);
#13614=EDGE_CURVE('',#11106,#11106,#10532,.T.);
#13615=EDGE_CURVE('',#11098,#11100,#10533,.T.);
#13616=EDGE_CURVE('',#11106,#11107,#4805,.T.);
#13617=EDGE_CURVE('',#11107,#11107,#10534,.T.);
#13618=EDGE_CURVE('',#11108,#11109,#119,.T.);
#13619=EDGE_CURVE('',#11109,#11110,#4806,.T.);
#13620=EDGE_CURVE('',#11110,#11111,#10535,.T.);
#13621=EDGE_CURVE('',#11111,#11110,#10536,.T.);
#13622=EDGE_CURVE('',#11109,#11112,#120,.T.);
#13623=EDGE_CURVE('',#11112,#11108,#10537,.T.);
#13624=EDGE_CURVE('',#11108,#11113,#4807,.T.);
#13625=EDGE_CURVE('',#11114,#11113,#121,.T.);
#13626=EDGE_CURVE('',#11115,#11114,#122,.T.);
#13627=EDGE_CURVE('',#11115,#11116,#4808,.T.);
#13628=EDGE_CURVE('',#11116,#11117,#4809,.T.);
#13629=EDGE_CURVE('',#11118,#11117,#4810,.T.);
#13630=EDGE_CURVE('',#11118,#11119,#4811,.T.);
#13631=EDGE_CURVE('',#11119,#11112,#4812,.T.);
#13632=EDGE_CURVE('',#11111,#11120,#4813,.T.);
#13633=EDGE_CURVE('',#11120,#11120,#10538,.T.);
#13634=EDGE_CURVE('',#11114,#11121,#4814,.T.);
#13635=EDGE_CURVE('',#11121,#11122,#10539,.T.);
#13636=EDGE_CURVE('',#11122,#11121,#10540,.T.);
#13637=EDGE_CURVE('',#11113,#11115,#10541,.T.);
#13638=EDGE_CURVE('',#11122,#11123,#4815,.T.);
#13639=EDGE_CURVE('',#11123,#11123,#10542,.T.);
#13640=EDGE_CURVE('',#11070,#11124,#4816,.T.);
#13641=EDGE_CURVE('',#11124,#11125,#10543,.T.);
#13642=EDGE_CURVE('',#11125,#11069,#4817,.T.);
#13643=EDGE_CURVE('',#11076,#11126,#4818,.T.);
#13644=EDGE_CURVE('',#11126,#11124,#4819,.T.);
#13645=EDGE_CURVE('',#11075,#11127,#4820,.T.);
#13646=EDGE_CURVE('',#11127,#11126,#10544,.T.);
#13647=EDGE_CURVE('',#11074,#11128,#4821,.T.);
#13648=EDGE_CURVE('',#11128,#11127,#4822,.T.);
#13649=EDGE_CURVE('',#11073,#11129,#4823,.T.);
#13650=EDGE_CURVE('',#11129,#11128,#10545,.T.);
#13651=EDGE_CURVE('',#11072,#11130,#4824,.T.);
#13652=EDGE_CURVE('',#11130,#11129,#4825,.T.);
#13653=EDGE_CURVE('',#11071,#11131,#4826,.T.);
#13654=EDGE_CURVE('',#11131,#11130,#10546,.T.);
#13655=EDGE_CURVE('',#11125,#11131,#4827,.T.);
#13656=EDGE_CURVE('',#11130,#11132,#4828,.T.);
#13657=EDGE_CURVE('',#11133,#11132,#4829,.T.);
#13658=EDGE_CURVE('',#11129,#11133,#4830,.T.);
#13659=EDGE_CURVE('',#11131,#11134,#4831,.T.);
#13660=EDGE_CURVE('',#11132,#11134,#10547,.T.);
#13661=EDGE_CURVE('',#11125,#11135,#4832,.T.);
#13662=EDGE_CURVE('',#11134,#11135,#4833,.T.);
#13663=EDGE_CURVE('',#11124,#11136,#4834,.T.);
#13664=EDGE_CURVE('',#11135,#11136,#10548,.T.);
#13665=EDGE_CURVE('',#11132,#11118,#4835,.T.);
#13666=EDGE_CURVE('',#11117,#11133,#4836,.T.);
#13667=EDGE_CURVE('',#11134,#11137,#4837,.T.);
#13668=EDGE_CURVE('',#11137,#11118,#10549,.T.);
#13669=EDGE_CURVE('',#11135,#11138,#4838,.T.);
#13670=EDGE_CURVE('',#11138,#11137,#4839,.T.);
#13671=EDGE_CURVE('',#11136,#11102,#4840,.T.);
#13672=EDGE_CURVE('',#11102,#11138,#10550,.T.);
#13673=EDGE_CURVE('',#11139,#11103,#4841,.T.);
#13674=EDGE_CURVE('',#11136,#11139,#4842,.T.);
#13675=EDGE_CURVE('',#11140,#11141,#4843,.T.);
#13676=EDGE_CURVE('',#11141,#11103,#10551,.T.);
#13677=EDGE_CURVE('',#11139,#11140,#10552,.T.);
#13678=EDGE_CURVE('',#11142,#11143,#4844,.T.);
#13679=EDGE_CURVE('',#11143,#11141,#4845,.T.);
#13680=EDGE_CURVE('',#11140,#11142,#4846,.T.);
#13681=EDGE_CURVE('',#11117,#11143,#10553,.T.);
#13682=EDGE_CURVE('',#11142,#11133,#10554,.T.);
#13683=EDGE_CURVE('',#11141,#11144,#4847,.T.);
#13684=EDGE_CURVE('',#11144,#11104,#10555,.T.);
#13685=EDGE_CURVE('',#11143,#11145,#4848,.T.);
#13686=EDGE_CURVE('',#11145,#11144,#4849,.T.);
#13687=EDGE_CURVE('',#11116,#11145,#10556,.T.);
#13688=EDGE_CURVE('',#11137,#11146,#4850,.T.);
#13689=EDGE_CURVE('',#11146,#11119,#10557,.T.);
#13690=EDGE_CURVE('',#11138,#11147,#4851,.T.);
#13691=EDGE_CURVE('',#11147,#11146,#4852,.T.);
#13692=EDGE_CURVE('',#11101,#11147,#10558,.T.);
#13693=EDGE_CURVE('',#11148,#11148,#10559,.T.);
#13694=EDGE_CURVE('',#11089,#11149,#4853,.T.);
#13695=EDGE_CURVE('',#11149,#11093,#10560,.T.);
#13696=EDGE_CURVE('',#11092,#11149,#4854,.T.);
#13697=EDGE_CURVE('',#11064,#11150,#4855,.T.);
#13698=EDGE_CURVE('',#11150,#11068,#10561,.T.);
#13699=EDGE_CURVE('',#11067,#11150,#4856,.T.);
#13700=EDGE_CURVE('',#11148,#11056,#4857,.T.);
#13701=EDGE_CURVE('',#11082,#11151,#4858,.T.);
#13702=EDGE_CURVE('',#11151,#11151,#10562,.T.);
#13703=EDGE_CURVE('',#11081,#11152,#4859,.T.);
#13704=EDGE_CURVE('',#11152,#11152,#10563,.T.);
#13705=EDGE_CURVE('',#11153,#11153,#10564,.T.);
#13706=EDGE_CURVE('',#11153,#11080,#4860,.T.);
#13707=EDGE_CURVE('',#11154,#11154,#10565,.T.);
#13708=EDGE_CURVE('',#11154,#11079,#4861,.T.);
#13709=EDGE_CURVE('',#11155,#11155,#10566,.T.);
#13710=EDGE_CURVE('',#11155,#11078,#4862,.T.);
#13711=EDGE_CURVE('',#11156,#11156,#10567,.T.);
#13712=EDGE_CURVE('',#11156,#11077,#4863,.T.);
#13713=EDGE_CURVE('',#11128,#11142,#4864,.T.);
#13714=EDGE_CURVE('',#11127,#11140,#4865,.T.);
#13715=EDGE_CURVE('',#11126,#11139,#4866,.T.);
#17582=ORIENTED_EDGE('',*,*,#13544,.T.);
#17583=ORIENTED_EDGE('',*,*,#13545,.T.);
#17584=ORIENTED_EDGE('',*,*,#13546,.T.);
#17585=ORIENTED_EDGE('',*,*,#13545,.F.);
#17586=ORIENTED_EDGE('',*,*,#13547,.F.);
#17587=ORIENTED_EDGE('',*,*,#13546,.F.);
#17588=ORIENTED_EDGE('',*,*,#13544,.F.);
#17589=ORIENTED_EDGE('',*,*,#13548,.T.);
#17590=ORIENTED_EDGE('',*,*,#13549,.T.);
#17591=ORIENTED_EDGE('',*,*,#13548,.F.);
#17592=ORIENTED_EDGE('',*,*,#13550,.T.);
#17593=ORIENTED_EDGE('',*,*,#13551,.T.);
#17594=ORIENTED_EDGE('',*,*,#13552,.T.);
#17595=ORIENTED_EDGE('',*,*,#13553,.T.);
#17596=ORIENTED_EDGE('',*,*,#13554,.T.);
#17597=ORIENTED_EDGE('',*,*,#13555,.T.);
#17598=ORIENTED_EDGE('',*,*,#13550,.F.);
#17599=ORIENTED_EDGE('',*,*,#13556,.T.);
#17600=ORIENTED_EDGE('',*,*,#13557,.T.);
#17601=ORIENTED_EDGE('',*,*,#13558,.T.);
#17602=ORIENTED_EDGE('',*,*,#13554,.F.);
#17603=ORIENTED_EDGE('',*,*,#13559,.T.);
#17604=ORIENTED_EDGE('',*,*,#13552,.F.);
#17605=ORIENTED_EDGE('',*,*,#13560,.T.);
#17606=ORIENTED_EDGE('',*,*,#13557,.F.);
#17607=ORIENTED_EDGE('',*,*,#13561,.T.);
#17608=ORIENTED_EDGE('',*,*,#13556,.F.);
#17609=ORIENTED_EDGE('',*,*,#13562,.T.);
#17610=ORIENTED_EDGE('',*,*,#13563,.T.);
#17611=ORIENTED_EDGE('',*,*,#13564,.F.);
#17612=ORIENTED_EDGE('',*,*,#13553,.F.);
#17613=ORIENTED_EDGE('',*,*,#13565,.T.);
#17614=ORIENTED_EDGE('',*,*,#13566,.T.);
#17615=ORIENTED_EDGE('',*,*,#13562,.F.);
#17616=ORIENTED_EDGE('',*,*,#13567,.F.);
#17617=ORIENTED_EDGE('',*,*,#13568,.F.);
#17618=ORIENTED_EDGE('',*,*,#13569,.F.);
#17619=ORIENTED_EDGE('',*,*,#13570,.F.);
#17620=ORIENTED_EDGE('',*,*,#13571,.F.);
#17621=ORIENTED_EDGE('',*,*,#13572,.F.);
#17622=ORIENTED_EDGE('',*,*,#13573,.F.);
#17623=ORIENTED_EDGE('',*,*,#13574,.F.);
#17624=ORIENTED_EDGE('',*,*,#13575,.T.);
#17625=ORIENTED_EDGE('',*,*,#13576,.T.);
#17626=ORIENTED_EDGE('',*,*,#13577,.T.);
#17627=ORIENTED_EDGE('',*,*,#13578,.T.);
#17628=ORIENTED_EDGE('',*,*,#13579,.T.);
#17629=ORIENTED_EDGE('',*,*,#13580,.T.);
#17630=ORIENTED_EDGE('',*,*,#13551,.F.);
#17631=ORIENTED_EDGE('',*,*,#13555,.F.);
#17632=ORIENTED_EDGE('',*,*,#13558,.F.);
#17633=ORIENTED_EDGE('',*,*,#13560,.F.);
#17634=ORIENTED_EDGE('',*,*,#13581,.T.);
#17635=ORIENTED_EDGE('',*,*,#13582,.T.);
#17636=ORIENTED_EDGE('',*,*,#13583,.T.);
#17637=ORIENTED_EDGE('',*,*,#13584,.T.);
#17638=ORIENTED_EDGE('',*,*,#13585,.T.);
#17639=ORIENTED_EDGE('',*,*,#13586,.T.);
#17640=ORIENTED_EDGE('',*,*,#13581,.F.);
#17641=ORIENTED_EDGE('',*,*,#13587,.T.);
#17642=ORIENTED_EDGE('',*,*,#13588,.T.);
#17643=ORIENTED_EDGE('',*,*,#13589,.T.);
#17644=ORIENTED_EDGE('',*,*,#13585,.F.);
#17645=ORIENTED_EDGE('',*,*,#13590,.T.);
#17646=ORIENTED_EDGE('',*,*,#13583,.F.);
#17647=ORIENTED_EDGE('',*,*,#13591,.T.);
#17648=ORIENTED_EDGE('',*,*,#13588,.F.);
#17649=ORIENTED_EDGE('',*,*,#13592,.T.);
#17650=ORIENTED_EDGE('',*,*,#13587,.F.);
#17651=ORIENTED_EDGE('',*,*,#13593,.T.);
#17652=ORIENTED_EDGE('',*,*,#13594,.T.);
#17653=ORIENTED_EDGE('',*,*,#13595,.F.);
#17654=ORIENTED_EDGE('',*,*,#13584,.F.);
#17655=ORIENTED_EDGE('',*,*,#13596,.T.);
#17656=ORIENTED_EDGE('',*,*,#13597,.T.);
#17657=ORIENTED_EDGE('',*,*,#13593,.F.);
#17658=ORIENTED_EDGE('',*,*,#13582,.F.);
#17659=ORIENTED_EDGE('',*,*,#13586,.F.);
#17660=ORIENTED_EDGE('',*,*,#13589,.F.);
#17661=ORIENTED_EDGE('',*,*,#13591,.F.);
#17662=ORIENTED_EDGE('',*,*,#13598,.T.);
#17663=ORIENTED_EDGE('',*,*,#13599,.T.);
#17664=ORIENTED_EDGE('',*,*,#13600,.T.);
#17665=ORIENTED_EDGE('',*,*,#13599,.F.);
#17666=ORIENTED_EDGE('',*,*,#13601,.T.);
#17667=ORIENTED_EDGE('',*,*,#13602,.T.);
#17668=ORIENTED_EDGE('',*,*,#13598,.F.);
#17669=ORIENTED_EDGE('',*,*,#13603,.T.);
#17670=ORIENTED_EDGE('',*,*,#13604,.F.);
#17671=ORIENTED_EDGE('',*,*,#13605,.F.);
#17672=ORIENTED_EDGE('',*,*,#13606,.T.);
#17673=ORIENTED_EDGE('',*,*,#13607,.F.);
#17674=ORIENTED_EDGE('',*,*,#13608,.F.);
#17675=ORIENTED_EDGE('',*,*,#13609,.T.);
#17676=ORIENTED_EDGE('',*,*,#13610,.T.);
#17677=ORIENTED_EDGE('',*,*,#13601,.F.);
#17678=ORIENTED_EDGE('',*,*,#13600,.F.);
#17679=ORIENTED_EDGE('',*,*,#13611,.T.);
#17680=ORIENTED_EDGE('',*,*,#13612,.T.);
#17681=ORIENTED_EDGE('',*,*,#13611,.F.);
#17682=ORIENTED_EDGE('',*,*,#13605,.T.);
#17683=ORIENTED_EDGE('',*,*,#13613,.T.);
#17684=ORIENTED_EDGE('',*,*,#13614,.T.);
#17685=ORIENTED_EDGE('',*,*,#13613,.F.);
#17686=ORIENTED_EDGE('',*,*,#13604,.T.);
#17687=ORIENTED_EDGE('',*,*,#13615,.T.);
#17688=ORIENTED_EDGE('',*,*,#13614,.F.);
#17689=ORIENTED_EDGE('',*,*,#13616,.T.);
#17690=ORIENTED_EDGE('',*,*,#13617,.T.);
#17691=ORIENTED_EDGE('',*,*,#13616,.F.);
#17692=ORIENTED_EDGE('',*,*,#13618,.T.);
#17693=ORIENTED_EDGE('',*,*,#13619,.T.);
#17694=ORIENTED_EDGE('',*,*,#13620,.T.);
#17695=ORIENTED_EDGE('',*,*,#13621,.T.);
#17696=ORIENTED_EDGE('',*,*,#13619,.F.);
#17697=ORIENTED_EDGE('',*,*,#13622,.T.);
#17698=ORIENTED_EDGE('',*,*,#13623,.T.);
#17699=ORIENTED_EDGE('',*,*,#13618,.F.);
#17700=ORIENTED_EDGE('',*,*,#13624,.T.);
#17701=ORIENTED_EDGE('',*,*,#13625,.F.);
#17702=ORIENTED_EDGE('',*,*,#13626,.F.);
#17703=ORIENTED_EDGE('',*,*,#13627,.T.);
#17704=ORIENTED_EDGE('',*,*,#13628,.T.);
#17705=ORIENTED_EDGE('',*,*,#13629,.F.);
#17706=ORIENTED_EDGE('',*,*,#13630,.T.);
#17707=ORIENTED_EDGE('',*,*,#13631,.T.);
#17708=ORIENTED_EDGE('',*,*,#13622,.F.);
#17709=ORIENTED_EDGE('',*,*,#13620,.F.);
#17710=ORIENTED_EDGE('',*,*,#13621,.F.);
#17711=ORIENTED_EDGE('',*,*,#13632,.T.);
#17712=ORIENTED_EDGE('',*,*,#13633,.T.);
#17713=ORIENTED_EDGE('',*,*,#13632,.F.);
#17714=ORIENTED_EDGE('',*,*,#13626,.T.);
#17715=ORIENTED_EDGE('',*,*,#13634,.T.);
#17716=ORIENTED_EDGE('',*,*,#13635,.T.);
#17717=ORIENTED_EDGE('',*,*,#13636,.T.);
#17718=ORIENTED_EDGE('',*,*,#13634,.F.);
#17719=ORIENTED_EDGE('',*,*,#13625,.T.);
#17720=ORIENTED_EDGE('',*,*,#13637,.T.);
#17721=ORIENTED_EDGE('',*,*,#13635,.F.);
#17722=ORIENTED_EDGE('',*,*,#13636,.F.);
#17723=ORIENTED_EDGE('',*,*,#13638,.T.);
#17724=ORIENTED_EDGE('',*,*,#13639,.T.);
#17725=ORIENTED_EDGE('',*,*,#13638,.F.);
#17726=ORIENTED_EDGE('',*,*,#13640,.T.);
#17727=ORIENTED_EDGE('',*,*,#13641,.T.);
#17728=ORIENTED_EDGE('',*,*,#13642,.T.);
#17729=ORIENTED_EDGE('',*,*,#13567,.T.);
#17730=ORIENTED_EDGE('',*,*,#13640,.F.);
#17731=ORIENTED_EDGE('',*,*,#13574,.T.);
#17732=ORIENTED_EDGE('',*,*,#13643,.T.);
#17733=ORIENTED_EDGE('',*,*,#13644,.T.);
#17734=ORIENTED_EDGE('',*,*,#13645,.T.);
#17735=ORIENTED_EDGE('',*,*,#13646,.T.);
#17736=ORIENTED_EDGE('',*,*,#13643,.F.);
#17737=ORIENTED_EDGE('',*,*,#13573,.T.);
#17738=ORIENTED_EDGE('',*,*,#13645,.F.);
#17739=ORIENTED_EDGE('',*,*,#13572,.T.);
#17740=ORIENTED_EDGE('',*,*,#13647,.T.);
#17741=ORIENTED_EDGE('',*,*,#13648,.T.);
#17742=ORIENTED_EDGE('',*,*,#13649,.T.);
#17743=ORIENTED_EDGE('',*,*,#13650,.T.);
#17744=ORIENTED_EDGE('',*,*,#13647,.F.);
#17745=ORIENTED_EDGE('',*,*,#13571,.T.);
#17746=ORIENTED_EDGE('',*,*,#13649,.F.);
#17747=ORIENTED_EDGE('',*,*,#13570,.T.);
#17748=ORIENTED_EDGE('',*,*,#13651,.T.);
#17749=ORIENTED_EDGE('',*,*,#13652,.T.);
#17750=ORIENTED_EDGE('',*,*,#13653,.T.);
#17751=ORIENTED_EDGE('',*,*,#13654,.T.);
#17752=ORIENTED_EDGE('',*,*,#13651,.F.);
#17753=ORIENTED_EDGE('',*,*,#13569,.T.);
#17754=ORIENTED_EDGE('',*,*,#13653,.F.);
#17755=ORIENTED_EDGE('',*,*,#13568,.T.);
#17756=ORIENTED_EDGE('',*,*,#13642,.F.);
#17757=ORIENTED_EDGE('',*,*,#13655,.T.);
#17758=ORIENTED_EDGE('',*,*,#13652,.F.);
#17759=ORIENTED_EDGE('',*,*,#13656,.T.);
#17760=ORIENTED_EDGE('',*,*,#13657,.F.);
#17761=ORIENTED_EDGE('',*,*,#13658,.F.);
#17762=ORIENTED_EDGE('',*,*,#13654,.F.);
#17763=ORIENTED_EDGE('',*,*,#13659,.T.);
#17764=ORIENTED_EDGE('',*,*,#13660,.F.);
#17765=ORIENTED_EDGE('',*,*,#13656,.F.);
#17766=ORIENTED_EDGE('',*,*,#13655,.F.);
#17767=ORIENTED_EDGE('',*,*,#13661,.T.);
#17768=ORIENTED_EDGE('',*,*,#13662,.F.);
#17769=ORIENTED_EDGE('',*,*,#13659,.F.);
#17770=ORIENTED_EDGE('',*,*,#13641,.F.);
#17771=ORIENTED_EDGE('',*,*,#13663,.T.);
#17772=ORIENTED_EDGE('',*,*,#13664,.F.);
#17773=ORIENTED_EDGE('',*,*,#13661,.F.);
#17774=ORIENTED_EDGE('',*,*,#13665,.T.);
#17775=ORIENTED_EDGE('',*,*,#13629,.T.);
#17776=ORIENTED_EDGE('',*,*,#13666,.T.);
#17777=ORIENTED_EDGE('',*,*,#13657,.T.);
#17778=ORIENTED_EDGE('',*,*,#13667,.T.);
#17779=ORIENTED_EDGE('',*,*,#13668,.T.);
#17780=ORIENTED_EDGE('',*,*,#13665,.F.);
#17781=ORIENTED_EDGE('',*,*,#13660,.T.);
#17782=ORIENTED_EDGE('',*,*,#13669,.T.);
#17783=ORIENTED_EDGE('',*,*,#13670,.T.);
#17784=ORIENTED_EDGE('',*,*,#13667,.F.);
#17785=ORIENTED_EDGE('',*,*,#13662,.T.);
#17786=ORIENTED_EDGE('',*,*,#13671,.T.);
#17787=ORIENTED_EDGE('',*,*,#13672,.T.);
#17788=ORIENTED_EDGE('',*,*,#13669,.F.);
#17789=ORIENTED_EDGE('',*,*,#13664,.T.);
#17790=ORIENTED_EDGE('',*,*,#13673,.T.);
#17791=ORIENTED_EDGE('',*,*,#13608,.T.);
#17792=ORIENTED_EDGE('',*,*,#13671,.F.);
#17793=ORIENTED_EDGE('',*,*,#13674,.T.);
#17794=ORIENTED_EDGE('',*,*,#13675,.T.);
#17795=ORIENTED_EDGE('',*,*,#13676,.T.);
#17796=ORIENTED_EDGE('',*,*,#13673,.F.);
#17797=ORIENTED_EDGE('',*,*,#13677,.T.);
#17798=ORIENTED_EDGE('',*,*,#13678,.T.);
#17799=ORIENTED_EDGE('',*,*,#13679,.T.);
#17800=ORIENTED_EDGE('',*,*,#13675,.F.);
#17801=ORIENTED_EDGE('',*,*,#13680,.T.);
#17802=ORIENTED_EDGE('',*,*,#13666,.F.);
#17803=ORIENTED_EDGE('',*,*,#13681,.T.);
#17804=ORIENTED_EDGE('',*,*,#13678,.F.);
#17805=ORIENTED_EDGE('',*,*,#13682,.T.);
#17806=ORIENTED_EDGE('',*,*,#13676,.F.);
#17807=ORIENTED_EDGE('',*,*,#13683,.T.);
#17808=ORIENTED_EDGE('',*,*,#13684,.T.);
#17809=ORIENTED_EDGE('',*,*,#13609,.F.);
#17810=ORIENTED_EDGE('',*,*,#13679,.F.);
#17811=ORIENTED_EDGE('',*,*,#13685,.T.);
#17812=ORIENTED_EDGE('',*,*,#13686,.T.);
#17813=ORIENTED_EDGE('',*,*,#13683,.F.);
#17814=ORIENTED_EDGE('',*,*,#13681,.F.);
#17815=ORIENTED_EDGE('',*,*,#13628,.F.);
#17816=ORIENTED_EDGE('',*,*,#13687,.T.);
#17817=ORIENTED_EDGE('',*,*,#13685,.F.);
#17818=ORIENTED_EDGE('',*,*,#13668,.F.);
#17819=ORIENTED_EDGE('',*,*,#13688,.T.);
#17820=ORIENTED_EDGE('',*,*,#13689,.T.);
#17821=ORIENTED_EDGE('',*,*,#13630,.F.);
#17822=ORIENTED_EDGE('',*,*,#13670,.F.);
#17823=ORIENTED_EDGE('',*,*,#13690,.T.);
#17824=ORIENTED_EDGE('',*,*,#13691,.T.);
#17825=ORIENTED_EDGE('',*,*,#13688,.F.);
#17826=ORIENTED_EDGE('',*,*,#13672,.F.);
#17827=ORIENTED_EDGE('',*,*,#13607,.T.);
#17828=ORIENTED_EDGE('',*,*,#13692,.T.);
#17829=ORIENTED_EDGE('',*,*,#13690,.F.);
#17830=ORIENTED_EDGE('',*,*,#13602,.F.);
#17831=ORIENTED_EDGE('',*,*,#13610,.F.);
#17832=ORIENTED_EDGE('',*,*,#13684,.F.);
#17833=ORIENTED_EDGE('',*,*,#13686,.F.);
#17834=ORIENTED_EDGE('',*,*,#13687,.F.);
#17835=ORIENTED_EDGE('',*,*,#13627,.F.);
#17836=ORIENTED_EDGE('',*,*,#13637,.F.);
#17837=ORIENTED_EDGE('',*,*,#13624,.F.);
#17838=ORIENTED_EDGE('',*,*,#13623,.F.);
#17839=ORIENTED_EDGE('',*,*,#13631,.F.);
#17840=ORIENTED_EDGE('',*,*,#13689,.F.);
#17841=ORIENTED_EDGE('',*,*,#13691,.F.);
#17842=ORIENTED_EDGE('',*,*,#13692,.F.);
#17843=ORIENTED_EDGE('',*,*,#13606,.F.);
#17844=ORIENTED_EDGE('',*,*,#13615,.F.);
#17845=ORIENTED_EDGE('',*,*,#13603,.F.);
#17846=ORIENTED_EDGE('',*,*,#13693,.T.);
#17847=ORIENTED_EDGE('',*,*,#13592,.F.);
#17848=ORIENTED_EDGE('',*,*,#13694,.T.);
#17849=ORIENTED_EDGE('',*,*,#13695,.T.);
#17850=ORIENTED_EDGE('',*,*,#13596,.F.);
#17851=ORIENTED_EDGE('',*,*,#13590,.F.);
#17852=ORIENTED_EDGE('',*,*,#13595,.T.);
#17853=ORIENTED_EDGE('',*,*,#13696,.T.);
#17854=ORIENTED_EDGE('',*,*,#13694,.F.);
#17855=ORIENTED_EDGE('',*,*,#13561,.F.);
#17856=ORIENTED_EDGE('',*,*,#13697,.T.);
#17857=ORIENTED_EDGE('',*,*,#13698,.T.);
#17858=ORIENTED_EDGE('',*,*,#13565,.F.);
#17859=ORIENTED_EDGE('',*,*,#13559,.F.);
#17860=ORIENTED_EDGE('',*,*,#13564,.T.);
#17861=ORIENTED_EDGE('',*,*,#13699,.T.);
#17862=ORIENTED_EDGE('',*,*,#13697,.F.);
#17863=ORIENTED_EDGE('',*,*,#13563,.F.);
#17864=ORIENTED_EDGE('',*,*,#13566,.F.);
#17865=ORIENTED_EDGE('',*,*,#13698,.F.);
#17866=ORIENTED_EDGE('',*,*,#13699,.F.);
#17867=ORIENTED_EDGE('',*,*,#13594,.F.);
#17868=ORIENTED_EDGE('',*,*,#13597,.F.);
#17869=ORIENTED_EDGE('',*,*,#13695,.F.);
#17870=ORIENTED_EDGE('',*,*,#13696,.F.);
#17871=ORIENTED_EDGE('',*,*,#13693,.F.);
#17872=ORIENTED_EDGE('',*,*,#13700,.T.);
#17873=ORIENTED_EDGE('',*,*,#13547,.T.);
#17874=ORIENTED_EDGE('',*,*,#13700,.F.);
#17875=ORIENTED_EDGE('',*,*,#13549,.F.);
#17876=ORIENTED_EDGE('',*,*,#13580,.F.);
#17877=ORIENTED_EDGE('',*,*,#13701,.T.);
#17878=ORIENTED_EDGE('',*,*,#13702,.T.);
#17879=ORIENTED_EDGE('',*,*,#13701,.F.);
#17880=ORIENTED_EDGE('',*,*,#13702,.F.);
#17881=ORIENTED_EDGE('',*,*,#13579,.F.);
#17882=ORIENTED_EDGE('',*,*,#13703,.T.);
#17883=ORIENTED_EDGE('',*,*,#13704,.T.);
#17884=ORIENTED_EDGE('',*,*,#13703,.F.);
#17885=ORIENTED_EDGE('',*,*,#13704,.F.);
#17886=ORIENTED_EDGE('',*,*,#13705,.F.);
#17887=ORIENTED_EDGE('',*,*,#13706,.T.);
#17888=ORIENTED_EDGE('',*,*,#13578,.F.);
#17889=ORIENTED_EDGE('',*,*,#13706,.F.);
#17890=ORIENTED_EDGE('',*,*,#13707,.F.);
#17891=ORIENTED_EDGE('',*,*,#13708,.T.);
#17892=ORIENTED_EDGE('',*,*,#13577,.F.);
#17893=ORIENTED_EDGE('',*,*,#13708,.F.);
#17894=ORIENTED_EDGE('',*,*,#13709,.F.);
#17895=ORIENTED_EDGE('',*,*,#13710,.T.);
#17896=ORIENTED_EDGE('',*,*,#13576,.F.);
#17897=ORIENTED_EDGE('',*,*,#13710,.F.);
#17898=ORIENTED_EDGE('',*,*,#13711,.F.);
#17899=ORIENTED_EDGE('',*,*,#13712,.T.);
#17900=ORIENTED_EDGE('',*,*,#13575,.F.);
#17901=ORIENTED_EDGE('',*,*,#13712,.F.);
#17902=ORIENTED_EDGE('',*,*,#13633,.F.);
#17903=ORIENTED_EDGE('',*,*,#13705,.T.);
#17904=ORIENTED_EDGE('',*,*,#13612,.F.);
#17905=ORIENTED_EDGE('',*,*,#13707,.T.);
#17906=ORIENTED_EDGE('',*,*,#13639,.F.);
#17907=ORIENTED_EDGE('',*,*,#13709,.T.);
#17908=ORIENTED_EDGE('',*,*,#13617,.F.);
#17909=ORIENTED_EDGE('',*,*,#13711,.T.);
#17910=ORIENTED_EDGE('',*,*,#13650,.F.);
#17911=ORIENTED_EDGE('',*,*,#13658,.T.);
#17912=ORIENTED_EDGE('',*,*,#13682,.F.);
#17913=ORIENTED_EDGE('',*,*,#13713,.F.);
#17914=ORIENTED_EDGE('',*,*,#13648,.F.);
#17915=ORIENTED_EDGE('',*,*,#13713,.T.);
#17916=ORIENTED_EDGE('',*,*,#13680,.F.);
#17917=ORIENTED_EDGE('',*,*,#13714,.F.);
#17918=ORIENTED_EDGE('',*,*,#13646,.F.);
#17919=ORIENTED_EDGE('',*,*,#13714,.T.);
#17920=ORIENTED_EDGE('',*,*,#13677,.F.);
#17921=ORIENTED_EDGE('',*,*,#13715,.F.);
#17922=ORIENTED_EDGE('',*,*,#13644,.F.);
#17923=ORIENTED_EDGE('',*,*,#13715,.T.);
#17924=ORIENTED_EDGE('',*,*,#13674,.F.);
#17925=ORIENTED_EDGE('',*,*,#13663,.F.);
#23568=CONICAL_SURFACE('',#25563,7.45,0.785398163397442);
#23569=CONICAL_SURFACE('',#25571,24.8,0.785398163397439);
#23570=CONICAL_SURFACE('',#25575,24.8,0.785398163397439);
#23571=CONICAL_SURFACE('',#25593,22.2,0.785398163397439);
#23572=CONICAL_SURFACE('',#25597,22.2,0.785398163397439);
#23573=CONICAL_SURFACE('',#25604,8.75,0.785398163397439);
#23574=CONICAL_SURFACE('',#25610,8.75,0.785398163397439);
#23575=CONICAL_SURFACE('',#25615,8.75,0.785398163397439);
#23576=CONICAL_SURFACE('',#25622,8.75,0.785398163397439);
#23577=CONICAL_SURFACE('',#25628,9.74999999999999,0.785398163397441);
#23578=CONICAL_SURFACE('',#25631,9.75,0.785398163397441);
#23579=CONICAL_SURFACE('',#25634,9.74999999999999,0.785398163397441);
#23580=CONICAL_SURFACE('',#25637,9.74999999999999,0.785398163397441);
#23581=CONICAL_SURFACE('',#25647,9.82322330470336,0.392699081698712);
#23582=CONICAL_SURFACE('',#25650,9.82322330470335,0.392699081698721);
#23583=CONICAL_SURFACE('',#25653,9.82322330470336,0.392699081698712);
#23584=CONICAL_SURFACE('',#25657,9.82322330470335,0.392699081698725);
#23585=CONICAL_SURFACE('',#25660,9.25,0.785398163397447);
#23586=CONICAL_SURFACE('',#25663,9.24999999999999,0.785398163397447);
#23587=CONICAL_SURFACE('',#25665,9.24999999999999,0.785398163397446);
#23588=CONICAL_SURFACE('',#25668,9.24999999999999,0.785398163397446);
#23834=ADVANCED_FACE('',(#1975),#23568,.F.);
#23835=ADVANCED_FACE('',(#1976,#631),#778,.T.);
#23836=ADVANCED_FACE('',(#1977),#494,.F.);
#23837=ADVANCED_FACE('',(#1978),#779,.T.);
#23838=ADVANCED_FACE('',(#1979),#23569,.F.);
#23839=ADVANCED_FACE('',(#1980),#780,.T.);
#23840=ADVANCED_FACE('',(#1981),#23570,.F.);
#23841=ADVANCED_FACE('',(#1982),#495,.F.);
#23842=ADVANCED_FACE('',(#1983),#781,.F.);
#23843=ADVANCED_FACE('',(#1984,#632,#633,#634,#635,#636,#637,#638),#782,
 .F.);
#23844=ADVANCED_FACE('',(#1985),#783,.T.);
#23845=ADVANCED_FACE('',(#1986),#23571,.T.);
#23846=ADVANCED_FACE('',(#1987),#784,.T.);
#23847=ADVANCED_FACE('',(#1988),#23572,.T.);
#23848=ADVANCED_FACE('',(#1989),#496,.T.);
#23849=ADVANCED_FACE('',(#1990),#785,.F.);
#23850=ADVANCED_FACE('',(#1991),#786,.F.);
#23851=ADVANCED_FACE('',(#1992),#23573,.F.);
#23852=ADVANCED_FACE('',(#1993),#787,.T.);
#23853=ADVANCED_FACE('',(#1994),#497,.F.);
#23854=ADVANCED_FACE('',(#1995),#23574,.F.);
#23855=ADVANCED_FACE('',(#1996),#498,.F.);
#23856=ADVANCED_FACE('',(#1997),#23575,.F.);
#23857=ADVANCED_FACE('',(#1998),#788,.T.);
#23858=ADVANCED_FACE('',(#1999),#499,.F.);
#23859=ADVANCED_FACE('',(#2000),#23576,.F.);
#23860=ADVANCED_FACE('',(#2001),#500,.F.);
#23861=ADVANCED_FACE('',(#2002),#23577,.T.);
#23862=ADVANCED_FACE('',(#2003),#789,.T.);
#23863=ADVANCED_FACE('',(#2004),#23578,.T.);
#23864=ADVANCED_FACE('',(#2005),#790,.T.);
#23865=ADVANCED_FACE('',(#2006),#23579,.T.);
#23866=ADVANCED_FACE('',(#2007),#791,.T.);
#23867=ADVANCED_FACE('',(#2008),#23580,.T.);
#23868=ADVANCED_FACE('',(#2009),#792,.T.);
#23869=ADVANCED_FACE('',(#2010),#793,.T.);
#23870=ADVANCED_FACE('',(#2011),#501,.T.);
#23871=ADVANCED_FACE('',(#2012),#794,.T.);
#23872=ADVANCED_FACE('',(#2013),#502,.T.);
#23873=ADVANCED_FACE('',(#2014),#795,.T.);
#23874=ADVANCED_FACE('',(#2015),#23581,.T.);
#23875=ADVANCED_FACE('',(#2016),#796,.T.);
#23876=ADVANCED_FACE('',(#2017),#23582,.T.);
#23877=ADVANCED_FACE('',(#2018),#797,.T.);
#23878=ADVANCED_FACE('',(#2019),#23583,.T.);
#23879=ADVANCED_FACE('',(#2020),#798,.T.);
#23880=ADVANCED_FACE('',(#2021),#23584,.T.);
#23881=ADVANCED_FACE('',(#2022),#23585,.T.);
#23882=ADVANCED_FACE('',(#2023),#799,.T.);
#23883=ADVANCED_FACE('',(#2024),#23586,.T.);
#23884=ADVANCED_FACE('',(#2025),#23587,.T.);
#23885=ADVANCED_FACE('',(#2026),#800,.T.);
#23886=ADVANCED_FACE('',(#2027),#23588,.T.);
#23887=ADVANCED_FACE('',(#2028,#639),#801,.T.);
#23888=ADVANCED_FACE('',(#2029),#503,.T.);
#23889=ADVANCED_FACE('',(#2030),#802,.F.);
#23890=ADVANCED_FACE('',(#2031),#504,.F.);
#23891=ADVANCED_FACE('',(#2032),#803,.F.);
#23892=ADVANCED_FACE('',(#2033,#640),#804,.F.);
#23893=ADVANCED_FACE('',(#2034),#505,.F.);
#23894=ADVANCED_FACE('',(#2035),#805,.T.);
#23895=ADVANCED_FACE('',(#2036),#506,.F.);
#23896=ADVANCED_FACE('',(#2037),#806,.F.);
#23897=ADVANCED_FACE('',(#2038),#507,.F.);
#23898=ADVANCED_FACE('',(#2039),#807,.F.);
#23899=ADVANCED_FACE('',(#2040),#508,.F.);
#23900=ADVANCED_FACE('',(#2041),#509,.F.);
#23901=ADVANCED_FACE('',(#2042),#510,.F.);
#23902=ADVANCED_FACE('',(#2043),#511,.F.);
#23903=ADVANCED_FACE('',(#2044,#641),#808,.T.);
#23904=ADVANCED_FACE('',(#2045,#642),#809,.T.);
#23905=ADVANCED_FACE('',(#2046,#643),#810,.T.);
#23906=ADVANCED_FACE('',(#2047,#644),#811,.T.);
#23907=ADVANCED_FACE('',(#2048),#512,.T.);
#23908=ADVANCED_FACE('',(#2049),#812,.T.);
#23909=ADVANCED_FACE('',(#2050),#513,.T.);
#23910=ADVANCED_FACE('',(#2051),#813,.T.);
#24939=CLOSED_SHELL('',(#23834,#23835,#23836,#23837,#23838,#23839,#23840,
#23841,#23842,#23843,#23844,#23845,#23846,#23847,#23848,#23849,#23850,#23851,
#23852,#23853,#23854,#23855,#23856,#23857,#23858,#23859,#23860,#23861,#23862,
#23863,#23864,#23865,#23866,#23867,#23868,#23869,#23870,#23871,#23872,#23873,
#23874,#23875,#23876,#23877,#23878,#23879,#23880,#23881,#23882,#23883,#23884,
#23885,#23886,#23887,#23888,#23889,#23890,#23891,#23892,#23893,#23894,#23895,
#23896,#23897,#23898,#23899,#23900,#23901,#23902,#23903,#23904,#23905,#23906,
#23907,#23908,#23909,#23910));
#25562=AXIS2_PLACEMENT_3D('',#35658,#28077,#28078);
#25563=AXIS2_PLACEMENT_3D('',#35659,#28079,#28080);
#25564=AXIS2_PLACEMENT_3D('',#35661,#28081,#28082);
#25565=AXIS2_PLACEMENT_3D('',#35664,#28084,#28085);
#25566=AXIS2_PLACEMENT_3D('',#35665,#28086,#28087);
#25567=AXIS2_PLACEMENT_3D('',#35667,#28088,#28089);
#25568=AXIS2_PLACEMENT_3D('',#35668,#28090,#28091);
#25569=AXIS2_PLACEMENT_3D('',#35671,#28093,#28094);
#25570=AXIS2_PLACEMENT_3D('',#35672,#28095,#28096);
#25571=AXIS2_PLACEMENT_3D('',#35681,#28101,#28102);
#25572=AXIS2_PLACEMENT_3D('',#35685,#28104,#28105);
#25573=AXIS2_PLACEMENT_3D('',#35686,#28106,#28107);
#25574=AXIS2_PLACEMENT_3D('',#35687,#28108,#28109);
#25575=AXIS2_PLACEMENT_3D('',#35693,#28113,#28114);
#25576=AXIS2_PLACEMENT_3D('',#35694,#28115,#28116);
#25577=AXIS2_PLACEMENT_3D('',#35695,#28117,#28118);
#25578=AXIS2_PLACEMENT_3D('',#35696,#28119,#28120);
#25579=AXIS2_PLACEMENT_3D('',#35700,#28122,#28123);
#25580=AXIS2_PLACEMENT_3D('',#35702,#28125,#28126);
#25581=AXIS2_PLACEMENT_3D('',#35706,#28129,#28130);
#25582=AXIS2_PLACEMENT_3D('',#35709,#28131,#28132);
#25583=AXIS2_PLACEMENT_3D('',#35713,#28134,#28135);
#25584=AXIS2_PLACEMENT_3D('',#35717,#28137,#28138);
#25585=AXIS2_PLACEMENT_3D('',#35721,#28140,#28141);
#25586=AXIS2_PLACEMENT_3D('',#35724,#28143,#28144);
#25587=AXIS2_PLACEMENT_3D('',#35726,#28145,#28146);
#25588=AXIS2_PLACEMENT_3D('',#35728,#28147,#28148);
#25589=AXIS2_PLACEMENT_3D('',#35730,#28149,#28150);
#25590=AXIS2_PLACEMENT_3D('',#35732,#28151,#28152);
#25591=AXIS2_PLACEMENT_3D('',#35734,#28153,#28154);
#25592=AXIS2_PLACEMENT_3D('',#35735,#28155,#28156);
#25593=AXIS2_PLACEMENT_3D('',#35744,#28161,#28162);
#25594=AXIS2_PLACEMENT_3D('',#35748,#28164,#28165);
#25595=AXIS2_PLACEMENT_3D('',#35749,#28166,#28167);
#25596=AXIS2_PLACEMENT_3D('',#35750,#28168,#28169);
#25597=AXIS2_PLACEMENT_3D('',#35756,#28173,#28174);
#25598=AXIS2_PLACEMENT_3D('',#35757,#28175,#28176);
#25599=AXIS2_PLACEMENT_3D('',#35758,#28177,#28178);
#25600=AXIS2_PLACEMENT_3D('',#35759,#28179,#28180);
#25601=AXIS2_PLACEMENT_3D('',#35763,#28182,#28183);
#25602=AXIS2_PLACEMENT_3D('',#35765,#28185,#28186);
#25603=AXIS2_PLACEMENT_3D('',#35769,#28189,#28190);
#25604=AXIS2_PLACEMENT_3D('',#35770,#28191,#28192);
#25605=AXIS2_PLACEMENT_3D('',#35778,#28194,#28195);
#25606=AXIS2_PLACEMENT_3D('',#35783,#28196,#28197);
#25607=AXIS2_PLACEMENT_3D('',#35784,#28198,#28199);
#25608=AXIS2_PLACEMENT_3D('',#35804,#28206,#28207);
#25609=AXIS2_PLACEMENT_3D('',#35807,#28209,#28210);
#25610=AXIS2_PLACEMENT_3D('',#35808,#28211,#28212);
#25611=AXIS2_PLACEMENT_3D('',#35811,#28214,#28215);
#25612=AXIS2_PLACEMENT_3D('',#35812,#28216,#28217);
#25613=AXIS2_PLACEMENT_3D('',#35813,#28218,#28219);
#25614=AXIS2_PLACEMENT_3D('',#35816,#28221,#28222);
#25615=AXIS2_PLACEMENT_3D('',#35817,#28223,#28224);
#25616=AXIS2_PLACEMENT_3D('',#35826,#28226,#28227);
#25617=AXIS2_PLACEMENT_3D('',#35827,#28228,#28229);
#25618=AXIS2_PLACEMENT_3D('',#35832,#28230,#28231);
#25619=AXIS2_PLACEMENT_3D('',#35833,#28232,#28233);
#25620=AXIS2_PLACEMENT_3D('',#35853,#28240,#28241);
#25621=AXIS2_PLACEMENT_3D('',#35856,#28243,#28244);
#25622=AXIS2_PLACEMENT_3D('',#35857,#28245,#28246);
#25623=AXIS2_PLACEMENT_3D('',#35861,#28248,#28249);
#25624=AXIS2_PLACEMENT_3D('',#35862,#28250,#28251);
#25625=AXIS2_PLACEMENT_3D('',#35863,#28252,#28253);
#25626=AXIS2_PLACEMENT_3D('',#35864,#28254,#28255);
#25627=AXIS2_PLACEMENT_3D('',#35867,#28257,#28258);
#25628=AXIS2_PLACEMENT_3D('',#35868,#28259,#28260);
#25629=AXIS2_PLACEMENT_3D('',#35872,#28262,#28263);
#25630=AXIS2_PLACEMENT_3D('',#35874,#28265,#28266);
#25631=AXIS2_PLACEMENT_3D('',#35878,#28269,#28270);
#25632=AXIS2_PLACEMENT_3D('',#35881,#28272,#28273);
#25633=AXIS2_PLACEMENT_3D('',#35882,#28274,#28275);
#25634=AXIS2_PLACEMENT_3D('',#35886,#28278,#28279);
#25635=AXIS2_PLACEMENT_3D('',#35889,#28281,#28282);
#25636=AXIS2_PLACEMENT_3D('',#35890,#28283,#28284);
#25637=AXIS2_PLACEMENT_3D('',#35894,#28287,#28288);
#25638=AXIS2_PLACEMENT_3D('',#35897,#28290,#28291);
#25639=AXIS2_PLACEMENT_3D('',#35898,#28292,#28293);
#25640=AXIS2_PLACEMENT_3D('',#35900,#28295,#28296);
#25641=AXIS2_PLACEMENT_3D('',#35906,#28300,#28301);
#25642=AXIS2_PLACEMENT_3D('',#35909,#28303,#28304);
#25643=AXIS2_PLACEMENT_3D('',#35910,#28305,#28306);
#25644=AXIS2_PLACEMENT_3D('',#35914,#28309,#28310);
#25645=AXIS2_PLACEMENT_3D('',#35917,#28312,#28313);
#25646=AXIS2_PLACEMENT_3D('',#35918,#28314,#28315);
#25647=AXIS2_PLACEMENT_3D('',#35921,#28318,#28319);
#25648=AXIS2_PLACEMENT_3D('',#35924,#28321,#28322);
#25649=AXIS2_PLACEMENT_3D('',#35925,#28323,#28324);
#25650=AXIS2_PLACEMENT_3D('',#35929,#28327,#28328);
#25651=AXIS2_PLACEMENT_3D('',#35931,#28330,#28331);
#25652=AXIS2_PLACEMENT_3D('',#35932,#28332,#28333);
#25653=AXIS2_PLACEMENT_3D('',#35936,#28336,#28337);
#25654=AXIS2_PLACEMENT_3D('',#35940,#28339,#28340);
#25655=AXIS2_PLACEMENT_3D('',#35941,#28341,#28342);
#25656=AXIS2_PLACEMENT_3D('',#35942,#28343,#28344);
#25657=AXIS2_PLACEMENT_3D('',#35948,#28348,#28349);
#25658=AXIS2_PLACEMENT_3D('',#35949,#28350,#28351);
#25659=AXIS2_PLACEMENT_3D('',#35950,#28352,#28353);
#25660=AXIS2_PLACEMENT_3D('',#35951,#28354,#28355);
#25661=AXIS2_PLACEMENT_3D('',#35954,#28357,#28358);
#25662=AXIS2_PLACEMENT_3D('',#35955,#28359,#28360);
#25663=AXIS2_PLACEMENT_3D('',#35959,#28363,#28364);
#25664=AXIS2_PLACEMENT_3D('',#35960,#28365,#28366);
#25665=AXIS2_PLACEMENT_3D('',#35961,#28367,#28368);
#25666=AXIS2_PLACEMENT_3D('',#35964,#28370,#28371);
#25667=AXIS2_PLACEMENT_3D('',#35965,#28372,#28373);
#25668=AXIS2_PLACEMENT_3D('',#35969,#28376,#28377);
#25669=AXIS2_PLACEMENT_3D('',#35970,#28378,#28379);
#25670=AXIS2_PLACEMENT_3D('',#35971,#28380,#28381);
#25671=AXIS2_PLACEMENT_3D('',#35973,#28382,#28383);
#25672=AXIS2_PLACEMENT_3D('',#35974,#28384,#28385);
#25673=AXIS2_PLACEMENT_3D('',#35977,#28387,#28388);
#25674=AXIS2_PLACEMENT_3D('',#35978,#28389,#28390);
#25675=AXIS2_PLACEMENT_3D('',#35980,#28392,#28393);
#25676=AXIS2_PLACEMENT_3D('',#35983,#28395,#28396);
#25677=AXIS2_PLACEMENT_3D('',#35984,#28397,#28398);
#25678=AXIS2_PLACEMENT_3D('',#35986,#28400,#28401);
#25679=AXIS2_PLACEMENT_3D('',#35987,#28402,#28403);
#25680=AXIS2_PLACEMENT_3D('',#35989,#28405,#28406);
#25681=AXIS2_PLACEMENT_3D('',#35990,#28407,#28408);
#25682=AXIS2_PLACEMENT_3D('',#35993,#28410,#28411);
#25683=AXIS2_PLACEMENT_3D('',#35994,#28412,#28413);
#25684=AXIS2_PLACEMENT_3D('',#35995,#28414,#28415);
#25685=AXIS2_PLACEMENT_3D('',#35998,#28417,#28418);
#25686=AXIS2_PLACEMENT_3D('',#35999,#28419,#28420);
#25687=AXIS2_PLACEMENT_3D('',#36000,#28421,#28422);
#25688=AXIS2_PLACEMENT_3D('',#36002,#28423,#28424);
#25689=AXIS2_PLACEMENT_3D('',#36004,#28426,#28427);
#25690=AXIS2_PLACEMENT_3D('',#36006,#28428,#28429);
#25691=AXIS2_PLACEMENT_3D('',#36008,#28431,#28432);
#25692=AXIS2_PLACEMENT_3D('',#36010,#28433,#28434);
#25693=AXIS2_PLACEMENT_3D('',#36012,#28436,#28437);
#25694=AXIS2_PLACEMENT_3D('',#36014,#28438,#28439);
#25695=AXIS2_PLACEMENT_3D('',#36016,#28441,#28442);
#25696=AXIS2_PLACEMENT_3D('',#36017,#28443,#28444);
#25697=AXIS2_PLACEMENT_3D('',#36018,#28445,#28446);
#25698=AXIS2_PLACEMENT_3D('',#36019,#28447,#28448);
#25699=AXIS2_PLACEMENT_3D('',#36020,#28449,#28450);
#25700=AXIS2_PLACEMENT_3D('',#36022,#28452,#28453);
#25701=AXIS2_PLACEMENT_3D('',#36024,#28455,#28456);
#25702=AXIS2_PLACEMENT_3D('',#36026,#28458,#28459);
#28077=DIRECTION('axis',(0.,0.,1.));
#28078=DIRECTION('refdir',(1.,0.,0.));
#28079=DIRECTION('center_axis',(0.,1.,0.));
#28080=DIRECTION('ref_axis',(1.,0.,0.));
#28081=DIRECTION('center_axis',(0.,-1.,0.));
#28082=DIRECTION('ref_axis',(1.,0.,0.));
#28083=DIRECTION('',(-0.707106781186543,0.707106781186552,-8.65956056235488E-17));
#28084=DIRECTION('center_axis',(0.,1.,0.));
#28085=DIRECTION('ref_axis',(1.,0.,0.));
#28086=DIRECTION('center_axis',(0.,1.,0.));
#28087=DIRECTION('ref_axis',(1.,0.,0.));
#28088=DIRECTION('center_axis',(0.,-1.,0.));
#28089=DIRECTION('ref_axis',(1.,0.,0.));
#28090=DIRECTION('center_axis',(0.,-1.,0.));
#28091=DIRECTION('ref_axis',(1.,0.,0.));
#28092=DIRECTION('',(0.,-1.,0.));
#28093=DIRECTION('center_axis',(0.,-1.,0.));
#28094=DIRECTION('ref_axis',(1.,0.,0.));
#28095=DIRECTION('center_axis',(0.707106781186554,-0.707106781186541,0.));
#28096=DIRECTION('ref_axis',(0.,0.,-1.));
#28097=DIRECTION('',(-0.707106781186541,-0.707106781186554,0.));
#28098=DIRECTION('',(0.,0.,-1.));
#28099=DIRECTION('',(0.707106781186541,0.707106781186554,0.));
#28100=DIRECTION('',(0.,0.,1.));
#28101=DIRECTION('center_axis',(0.,-1.,0.));
#28102=DIRECTION('ref_axis',(-1.,0.,0.));
#28103=DIRECTION('',(0.707106781186541,-0.707106781186554,8.65956056235483E-17));
#28104=DIRECTION('center_axis',(0.,-1.,0.));
#28105=DIRECTION('ref_axis',(-1.,0.,0.));
#28106=DIRECTION('center_axis',(0.,1.,0.));
#28107=DIRECTION('ref_axis',(-1.,0.,0.));
#28108=DIRECTION('center_axis',(-0.707106781186554,-0.707106781186541,0.));
#28109=DIRECTION('ref_axis',(0.,0.,1.));
#28110=DIRECTION('',(0.707106781186541,-0.707106781186554,0.));
#28111=DIRECTION('',(0.,0.,1.));
#28112=DIRECTION('',(0.,0.,-1.));
#28113=DIRECTION('center_axis',(0.,-1.,0.));
#28114=DIRECTION('ref_axis',(1.,0.,0.));
#28115=DIRECTION('center_axis',(0.,-1.,0.));
#28116=DIRECTION('ref_axis',(1.,0.,0.));
#28117=DIRECTION('center_axis',(0.,1.,0.));
#28118=DIRECTION('ref_axis',(1.,0.,0.));
#28119=DIRECTION('center_axis',(0.,1.,0.));
#28120=DIRECTION('ref_axis',(-1.,0.,0.));
#28121=DIRECTION('',(0.,1.,0.));
#28122=DIRECTION('center_axis',(0.,1.,0.));
#28123=DIRECTION('ref_axis',(-1.,0.,0.));
#28124=DIRECTION('',(0.,1.,0.));
#28125=DIRECTION('center_axis',(-1.,0.,0.));
#28126=DIRECTION('ref_axis',(0.,0.,1.));
#28127=DIRECTION('',(0.,1.,0.));
#28128=DIRECTION('',(0.,0.,1.));
#28129=DIRECTION('center_axis',(0.,1.,0.));
#28130=DIRECTION('ref_axis',(1.,0.,0.));
#28131=DIRECTION('center_axis',(0.,1.,0.));
#28132=DIRECTION('ref_axis',(1.33226762955019E-15,0.,-1.));
#28133=DIRECTION('',(-1.,0.,0.));
#28134=DIRECTION('center_axis',(0.,1.,0.));
#28135=DIRECTION('ref_axis',(1.,0.,8.88178419700126E-16));
#28136=DIRECTION('',(0.,0.,-1.));
#28137=DIRECTION('center_axis',(0.,1.,0.));
#28138=DIRECTION('ref_axis',(-4.44089209850063E-16,0.,1.));
#28139=DIRECTION('',(1.,0.,0.));
#28140=DIRECTION('center_axis',(0.,1.,0.));
#28141=DIRECTION('ref_axis',(-1.,0.,-8.88178419700126E-16));
#28142=DIRECTION('',(0.,0.,1.));
#28143=DIRECTION('center_axis',(0.,1.,0.));
#28144=DIRECTION('ref_axis',(1.,0.,0.));
#28145=DIRECTION('center_axis',(0.,1.,0.));
#28146=DIRECTION('ref_axis',(1.,0.,0.));
#28147=DIRECTION('center_axis',(0.,1.,0.));
#28148=DIRECTION('ref_axis',(1.,0.,0.));
#28149=DIRECTION('center_axis',(0.,1.,0.));
#28150=DIRECTION('ref_axis',(1.,0.,0.));
#28151=DIRECTION('center_axis',(0.,1.,0.));
#28152=DIRECTION('ref_axis',(1.,0.,0.));
#28153=DIRECTION('center_axis',(0.,1.,0.));
#28154=DIRECTION('ref_axis',(1.,0.,0.));
#28155=DIRECTION('center_axis',(0.707106781186554,-0.707106781186541,0.));
#28156=DIRECTION('ref_axis',(0.,0.,-1.));
#28157=DIRECTION('',(-0.707106781186541,-0.707106781186554,2.39222714223772E-15));
#28158=DIRECTION('',(0.,0.,-1.));
#28159=DIRECTION('',(0.707106781186541,0.707106781186554,0.));
#28160=DIRECTION('',(0.,0.,1.));
#28161=DIRECTION('center_axis',(0.,1.,0.));
#28162=DIRECTION('ref_axis',(-1.,0.,0.));
#28163=DIRECTION('',(0.707106781186541,-0.707106781186554,7.60309417374759E-15));
#28164=DIRECTION('center_axis',(0.,1.,0.));
#28165=DIRECTION('ref_axis',(-1.,0.,0.));
#28166=DIRECTION('center_axis',(0.,-1.,0.));
#28167=DIRECTION('ref_axis',(-1.,0.,0.));
#28168=DIRECTION('center_axis',(-0.707106781186554,-0.707106781186541,0.));
#28169=DIRECTION('ref_axis',(0.,0.,1.));
#28170=DIRECTION('',(0.707106781186541,-0.707106781186554,0.));
#28171=DIRECTION('',(0.,0.,1.));
#28172=DIRECTION('',(0.,0.,-1.));
#28173=DIRECTION('center_axis',(0.,1.,0.));
#28174=DIRECTION('ref_axis',(1.,0.,-1.97812565634772E-16));
#28175=DIRECTION('center_axis',(0.,1.,0.));
#28176=DIRECTION('ref_axis',(1.,0.,-1.97812565634772E-16));
#28177=DIRECTION('center_axis',(0.,-1.,0.));
#28178=DIRECTION('ref_axis',(1.,0.,-1.97812565634772E-16));
#28179=DIRECTION('center_axis',(0.,1.,0.));
#28180=DIRECTION('ref_axis',(-1.,0.,0.));
#28181=DIRECTION('',(0.,1.,0.));
#28182=DIRECTION('center_axis',(0.,-1.,0.));
#28183=DIRECTION('ref_axis',(-1.,0.,0.));
#28184=DIRECTION('',(0.,1.,0.));
#28185=DIRECTION('center_axis',(-1.,0.,0.));
#28186=DIRECTION('ref_axis',(0.,0.,1.));
#28187=DIRECTION('',(0.,1.,0.));
#28188=DIRECTION('',(0.,0.,1.));
#28189=DIRECTION('center_axis',(0.,1.,0.));
#28190=DIRECTION('ref_axis',(1.,0.,0.));
#28191=DIRECTION('center_axis',(0.,1.,0.));
#28192=DIRECTION('ref_axis',(1.,0.,0.));
#28193=DIRECTION('',(0.707106781186541,-0.707106781186554,-8.65956056235486E-17));
#28194=DIRECTION('center_axis',(0.,-1.,0.));
#28195=DIRECTION('ref_axis',(1.,0.,0.));
#28196=DIRECTION('center_axis',(0.,1.,0.));
#28197=DIRECTION('ref_axis',(1.,0.,0.));
#28198=DIRECTION('center_axis',(-0.707106781186549,0.707106781186546,0.));
#28199=DIRECTION('ref_axis',(0.,0.,1.));
#28200=DIRECTION('',(0.,0.,-1.));
#28201=DIRECTION('',(0.,0.,-1.));
#28202=DIRECTION('',(0.707106781186548,0.707106781186548,0.));
#28203=DIRECTION('',(0.,0.,-1.));
#28204=DIRECTION('',(0.707106781186546,0.707106781186549,0.));
#28205=DIRECTION('',(0.,0.,-1.));
#28206=DIRECTION('center_axis',(0.,-1.,0.));
#28207=DIRECTION('ref_axis',(1.,0.,0.));
#28208=DIRECTION('',(0.,-1.,0.));
#28209=DIRECTION('center_axis',(0.,-1.,0.));
#28210=DIRECTION('ref_axis',(1.,0.,0.));
#28211=DIRECTION('center_axis',(0.,1.,0.));
#28212=DIRECTION('ref_axis',(1.,0.,0.));
#28213=DIRECTION('',(0.707106781186541,-0.707106781186554,-8.65956056235486E-17));
#28214=DIRECTION('center_axis',(0.,-1.,0.));
#28215=DIRECTION('ref_axis',(1.,0.,0.));
#28216=DIRECTION('center_axis',(0.,1.,0.));
#28217=DIRECTION('ref_axis',(1.,0.,0.));
#28218=DIRECTION('center_axis',(0.,-1.,0.));
#28219=DIRECTION('ref_axis',(1.,0.,0.));
#28220=DIRECTION('',(0.,-1.,0.));
#28221=DIRECTION('center_axis',(0.,-1.,0.));
#28222=DIRECTION('ref_axis',(1.,0.,0.));
#28223=DIRECTION('center_axis',(0.,1.,0.));
#28224=DIRECTION('ref_axis',(-1.,0.,0.));
#28225=DIRECTION('',(-0.707106781186541,-0.707106781186554,8.65956056235486E-17));
#28226=DIRECTION('center_axis',(0.,-1.,0.));
#28227=DIRECTION('ref_axis',(-1.,0.,0.));
#28228=DIRECTION('center_axis',(0.,-1.,0.));
#28229=DIRECTION('ref_axis',(-1.,0.,0.));
#28230=DIRECTION('center_axis',(0.,1.,0.));
#28231=DIRECTION('ref_axis',(-1.,0.,0.));
#28232=DIRECTION('center_axis',(0.707106781186549,0.707106781186546,0.));
#28233=DIRECTION('ref_axis',(0.,0.,-1.));
#28234=DIRECTION('',(0.,0.,1.));
#28235=DIRECTION('',(0.,0.,1.));
#28236=DIRECTION('',(0.707106781186544,-0.707106781186551,0.));
#28237=DIRECTION('',(0.,0.,1.));
#28238=DIRECTION('',(-0.707106781186546,0.707106781186549,0.));
#28239=DIRECTION('',(0.,0.,1.));
#28240=DIRECTION('center_axis',(0.,-1.,0.));
#28241=DIRECTION('ref_axis',(1.,0.,0.));
#28242=DIRECTION('',(0.,-1.,0.));
#28243=DIRECTION('center_axis',(0.,-1.,0.));
#28244=DIRECTION('ref_axis',(1.,0.,0.));
#28245=DIRECTION('center_axis',(0.,1.,0.));
#28246=DIRECTION('ref_axis',(-1.,0.,0.));
#28247=DIRECTION('',(-0.707106781186541,-0.707106781186554,8.65956056235486E-17));
#28248=DIRECTION('center_axis',(0.,-1.,0.));
#28249=DIRECTION('ref_axis',(-1.,0.,0.));
#28250=DIRECTION('center_axis',(0.,-1.,0.));
#28251=DIRECTION('ref_axis',(-1.,0.,0.));
#28252=DIRECTION('center_axis',(0.,1.,0.));
#28253=DIRECTION('ref_axis',(-1.,0.,0.));
#28254=DIRECTION('center_axis',(0.,-1.,0.));
#28255=DIRECTION('ref_axis',(1.,0.,0.));
#28256=DIRECTION('',(0.,-1.,0.));
#28257=DIRECTION('center_axis',(0.,-1.,0.));
#28258=DIRECTION('ref_axis',(1.,0.,0.));
#28259=DIRECTION('center_axis',(0.,1.,0.));
#28260=DIRECTION('ref_axis',(1.33226762955019E-15,0.,-1.));
#28261=DIRECTION('',(-0.707106781186547,0.707106781186547,0.));
#28262=DIRECTION('center_axis',(0.,-1.,0.));
#28263=DIRECTION('ref_axis',(1.33226762955019E-15,0.,-1.));
#28264=DIRECTION('',(0.,-0.707106781186554,0.707106781186541));
#28265=DIRECTION('center_axis',(-0.707106781186554,-0.707106781186541,0.));
#28266=DIRECTION('ref_axis',(0.,0.,1.));
#28267=DIRECTION('',(-0.707106781186541,0.707106781186554,0.));
#28268=DIRECTION('',(0.,0.,-1.));
#28269=DIRECTION('center_axis',(0.,1.,0.));
#28270=DIRECTION('ref_axis',(-1.,0.,-8.88178419700126E-16));
#28271=DIRECTION('',(0.,0.707106781186554,0.707106781186541));
#28272=DIRECTION('center_axis',(0.,-1.,0.));
#28273=DIRECTION('ref_axis',(-1.,0.,-8.88178419700126E-16));
#28274=DIRECTION('center_axis',(0.,-0.707106781186541,0.707106781186554));
#28275=DIRECTION('ref_axis',(1.,0.,0.));
#28276=DIRECTION('',(6.28036983473507E-15,0.707106781186554,0.707106781186541));
#28277=DIRECTION('',(-1.,0.,0.));
#28278=DIRECTION('center_axis',(0.,1.,0.));
#28279=DIRECTION('ref_axis',(-4.44089209850063E-16,0.,1.));
#28280=DIRECTION('',(0.707106781186538,0.707106781186557,0.));
#28281=DIRECTION('center_axis',(0.,-1.,0.));
#28282=DIRECTION('ref_axis',(-4.44089209850063E-16,0.,1.));
#28283=DIRECTION('center_axis',(0.707106781186554,-0.707106781186541,0.));
#28284=DIRECTION('ref_axis',(0.,0.,-1.));
#28285=DIRECTION('',(0.707106781186541,0.707106781186554,0.));
#28286=DIRECTION('',(0.,0.,1.));
#28287=DIRECTION('center_axis',(0.,1.,0.));
#28288=DIRECTION('ref_axis',(1.,0.,8.88178419700126E-16));
#28289=DIRECTION('',(0.,0.707106781186554,-0.707106781186541));
#28290=DIRECTION('center_axis',(0.,-1.,0.));
#28291=DIRECTION('ref_axis',(1.,0.,8.88178419700126E-16));
#28292=DIRECTION('center_axis',(0.,-0.707106781186541,-0.707106781186554));
#28293=DIRECTION('ref_axis',(-1.,0.,0.));
#28294=DIRECTION('',(1.,0.,0.));
#28295=DIRECTION('center_axis',(1.,0.,0.));
#28296=DIRECTION('ref_axis',(0.,0.,-1.));
#28297=DIRECTION('',(0.,1.,0.));
#28298=DIRECTION('',(0.,0.,-1.));
#28299=DIRECTION('',(0.,1.,0.));
#28300=DIRECTION('center_axis',(0.,1.,0.));
#28301=DIRECTION('ref_axis',(1.,0.,8.88178419700126E-16));
#28302=DIRECTION('',(0.,1.,0.));
#28303=DIRECTION('center_axis',(0.,1.,0.));
#28304=DIRECTION('ref_axis',(1.,0.,8.88178419700126E-16));
#28305=DIRECTION('center_axis',(0.,0.,-1.));
#28306=DIRECTION('ref_axis',(-1.,0.,0.));
#28307=DIRECTION('',(0.,1.,0.));
#28308=DIRECTION('',(-1.,0.,0.));
#28309=DIRECTION('center_axis',(0.,1.,0.));
#28310=DIRECTION('ref_axis',(1.33226762955019E-15,0.,-1.));
#28311=DIRECTION('',(0.,1.,0.));
#28312=DIRECTION('center_axis',(0.,1.,0.));
#28313=DIRECTION('ref_axis',(1.33226762955019E-15,0.,-1.));
#28314=DIRECTION('center_axis',(0.923879532511288,0.382683432365087,0.));
#28315=DIRECTION('ref_axis',(0.,0.,-1.));
#28316=DIRECTION('',(-0.382683432365087,0.923879532511288,0.));
#28317=DIRECTION('',(0.382683432365078,-0.923879532511291,0.));
#28318=DIRECTION('center_axis',(5.20282872453227E-15,-1.,0.));
#28319=DIRECTION('ref_axis',(1.,0.,9.04161894879113E-16));
#28320=DIRECTION('',(0.,0.923879532511288,0.382683432365087));
#28321=DIRECTION('center_axis',(0.,-1.,0.));
#28322=DIRECTION('ref_axis',(1.,0.,9.20731182852366E-16));
#28323=DIRECTION('center_axis',(0.,0.382683432365087,-0.923879532511288));
#28324=DIRECTION('ref_axis',(-1.,0.,0.));
#28325=DIRECTION('',(0.,0.923879532511282,0.382683432365102));
#28326=DIRECTION('',(1.,0.,0.));
#28327=DIRECTION('center_axis',(0.,-1.,0.));
#28328=DIRECTION('ref_axis',(1.35624284231867E-15,0.,-1.));
#28329=DIRECTION('',(0.382683432365103,0.923879532511281,0.));
#28330=DIRECTION('center_axis',(0.,-1.,0.));
#28331=DIRECTION('ref_axis',(1.38109677427855E-15,0.,-1.));
#28332=DIRECTION('center_axis',(-0.923879532511288,0.382683432365087,0.));
#28333=DIRECTION('ref_axis',(0.,0.,1.));
#28334=DIRECTION('',(0.382683432365087,0.923879532511288,0.));
#28335=DIRECTION('',(0.,0.,1.));
#28336=DIRECTION('center_axis',(0.,-1.,0.));
#28337=DIRECTION('ref_axis',(-1.,0.,-9.04161894879113E-16));
#28338=DIRECTION('',(0.,0.923879532511288,-0.382683432365087));
#28339=DIRECTION('center_axis',(0.,-1.,0.));
#28340=DIRECTION('ref_axis',(-1.,0.,-9.20731182852366E-16));
#28341=DIRECTION('center_axis',(0.,1.,0.));
#28342=DIRECTION('ref_axis',(-1.,0.,-8.88178419700126E-16));
#28343=DIRECTION('center_axis',(0.,0.382683432365083,0.92387953251129));
#28344=DIRECTION('ref_axis',(1.,0.,0.));
#28345=DIRECTION('',(0.,0.92387953251129,-0.382683432365083));
#28346=DIRECTION('',(-1.,0.,0.));
#28347=DIRECTION('',(1.,0.,0.));
#28348=DIRECTION('center_axis',(0.,-1.,0.));
#28349=DIRECTION('ref_axis',(-4.52080947439557E-16,0.,1.));
#28350=DIRECTION('center_axis',(0.,-1.,0.));
#28351=DIRECTION('ref_axis',(-4.60365591426184E-16,0.,1.));
#28352=DIRECTION('center_axis',(0.,1.,0.));
#28353=DIRECTION('ref_axis',(-4.44089209850063E-16,0.,1.));
#28354=DIRECTION('center_axis',(0.,-1.,0.));
#28355=DIRECTION('ref_axis',(-1.,0.,-8.88178419700126E-16));
#28356=DIRECTION('',(-2.09345661157836E-15,0.707106781186549,-0.707106781186546));
#28357=DIRECTION('center_axis',(0.,-1.,0.));
#28358=DIRECTION('ref_axis',(-1.,0.,-8.88178419700126E-16));
#28359=DIRECTION('center_axis',(0.,0.707106781186546,0.707106781186549));
#28360=DIRECTION('ref_axis',(1.,0.,0.));
#28361=DIRECTION('',(-2.09345661157836E-15,0.707106781186549,-0.707106781186546));
#28362=DIRECTION('',(-1.,0.,0.));
#28363=DIRECTION('center_axis',(0.,-1.,0.));
#28364=DIRECTION('ref_axis',(-4.44089209850063E-16,0.,1.));
#28365=DIRECTION('center_axis',(0.,-1.,0.));
#28366=DIRECTION('ref_axis',(-4.44089209850063E-16,0.,1.));
#28367=DIRECTION('center_axis',(0.,-1.,0.));
#28368=DIRECTION('ref_axis',(1.,0.,8.88178419700126E-16));
#28369=DIRECTION('',(2.09345661157837E-15,0.70710678118655,0.707106781186545));
#28370=DIRECTION('center_axis',(0.,-1.,0.));
#28371=DIRECTION('ref_axis',(1.,0.,8.88178419700126E-16));
#28372=DIRECTION('center_axis',(0.,0.707106781186548,-0.707106781186548));
#28373=DIRECTION('ref_axis',(-1.,0.,0.));
#28374=DIRECTION('',(2.09345661157836E-15,0.707106781186548,0.707106781186548));
#28375=DIRECTION('',(1.,0.,0.));
#28376=DIRECTION('center_axis',(0.,-1.,0.));
#28377=DIRECTION('ref_axis',(1.33226762955019E-15,0.,-1.));
#28378=DIRECTION('center_axis',(0.,-1.,0.));
#28379=DIRECTION('ref_axis',(1.33226762955019E-15,0.,-1.));
#28380=DIRECTION('center_axis',(0.,1.,0.));
#28381=DIRECTION('ref_axis',(1.,0.,0.));
#28382=DIRECTION('center_axis',(0.,-1.,0.));
#28383=DIRECTION('ref_axis',(1.,0.,0.));
#28384=DIRECTION('center_axis',(0.,1.,0.));
#28385=DIRECTION('ref_axis',(1.,0.,-1.97812565634772E-16));
#28386=DIRECTION('',(0.,1.,0.));
#28387=DIRECTION('center_axis',(0.,-1.,0.));
#28388=DIRECTION('ref_axis',(1.,0.,-1.97812565634772E-16));
#28389=DIRECTION('center_axis',(1.,0.,0.));
#28390=DIRECTION('ref_axis',(0.,0.,-1.));
#28391=DIRECTION('',(0.,0.,-1.));
#28392=DIRECTION('center_axis',(0.,1.,0.));
#28393=DIRECTION('ref_axis',(1.,0.,0.));
#28394=DIRECTION('',(0.,1.,0.));
#28395=DIRECTION('center_axis',(0.,1.,0.));
#28396=DIRECTION('ref_axis',(1.,0.,0.));
#28397=DIRECTION('center_axis',(1.,0.,0.));
#28398=DIRECTION('ref_axis',(0.,0.,-1.));
#28399=DIRECTION('',(0.,0.,-1.));
#28400=DIRECTION('center_axis',(0.,1.,0.));
#28401=DIRECTION('ref_axis',(1.,0.,0.));
#28402=DIRECTION('center_axis',(0.,-1.,0.));
#28403=DIRECTION('ref_axis',(1.,0.,0.));
#28404=DIRECTION('',(0.,-1.,0.));
#28405=DIRECTION('center_axis',(0.,1.,0.));
#28406=DIRECTION('ref_axis',(1.,0.,0.));
#28407=DIRECTION('center_axis',(0.,1.,0.));
#28408=DIRECTION('ref_axis',(1.,0.,0.));
#28409=DIRECTION('',(0.,1.,0.));
#28410=DIRECTION('center_axis',(0.,1.,0.));
#28411=DIRECTION('ref_axis',(1.,0.,0.));
#28412=DIRECTION('center_axis',(0.,1.,0.));
#28413=DIRECTION('ref_axis',(1.,0.,0.));
#28414=DIRECTION('center_axis',(0.,1.,0.));
#28415=DIRECTION('ref_axis',(1.,0.,0.));
#28416=DIRECTION('',(0.,1.,0.));
#28417=DIRECTION('center_axis',(0.,1.,0.));
#28418=DIRECTION('ref_axis',(1.,0.,0.));
#28419=DIRECTION('center_axis',(0.,1.,0.));
#28420=DIRECTION('ref_axis',(1.,0.,0.));
#28421=DIRECTION('center_axis',(0.,-1.,0.));
#28422=DIRECTION('ref_axis',(1.,0.,0.));
#28423=DIRECTION('center_axis',(0.,-1.,0.));
#28424=DIRECTION('ref_axis',(1.,0.,0.));
#28425=DIRECTION('',(0.,-1.,0.));
#28426=DIRECTION('center_axis',(0.,-1.,0.));
#28427=DIRECTION('ref_axis',(1.,0.,0.));
#28428=DIRECTION('center_axis',(0.,-1.,0.));
#28429=DIRECTION('ref_axis',(1.,0.,0.));
#28430=DIRECTION('',(0.,-1.,0.));
#28431=DIRECTION('center_axis',(0.,-1.,0.));
#28432=DIRECTION('ref_axis',(1.,0.,0.));
#28433=DIRECTION('center_axis',(0.,-1.,0.));
#28434=DIRECTION('ref_axis',(1.,0.,0.));
#28435=DIRECTION('',(0.,-1.,0.));
#28436=DIRECTION('center_axis',(0.,-1.,0.));
#28437=DIRECTION('ref_axis',(1.,0.,0.));
#28438=DIRECTION('center_axis',(0.,-1.,0.));
#28439=DIRECTION('ref_axis',(1.,0.,0.));
#28440=DIRECTION('',(0.,-1.,0.));
#28441=DIRECTION('center_axis',(0.,1.,0.));
#28442=DIRECTION('ref_axis',(1.,0.,0.));
#28443=DIRECTION('center_axis',(0.,1.,0.));
#28444=DIRECTION('ref_axis',(1.,0.,0.));
#28445=DIRECTION('center_axis',(0.,1.,0.));
#28446=DIRECTION('ref_axis',(1.,0.,0.));
#28447=DIRECTION('center_axis',(0.,1.,0.));
#28448=DIRECTION('ref_axis',(1.,0.,0.));
#28449=DIRECTION('center_axis',(0.,1.,0.));
#28450=DIRECTION('ref_axis',(-4.44089209850063E-16,0.,1.));
#28451=DIRECTION('',(0.,1.,0.));
#28452=DIRECTION('center_axis',(0.,0.,1.));
#28453=DIRECTION('ref_axis',(1.,0.,0.));
#28454=DIRECTION('',(0.,1.,0.));
#28455=DIRECTION('center_axis',(0.,1.,0.));
#28456=DIRECTION('ref_axis',(-1.,0.,-8.88178419700126E-16));
#28457=DIRECTION('',(0.,1.,0.));
#28458=DIRECTION('center_axis',(-1.,0.,0.));
#28459=DIRECTION('ref_axis',(0.,0.,1.));
#35658=CARTESIAN_POINT('',(0.,0.,0.));
#35659=CARTESIAN_POINT('Origin',(0.,105.05,-16.5));
#35660=CARTESIAN_POINT('',(-7.2,104.8,-16.5));
#35661=CARTESIAN_POINT('Origin',(0.,104.8,-16.5));
#35662=CARTESIAN_POINT('',(-7.7,105.3,-16.5));
#35663=CARTESIAN_POINT('',(-7.45,105.05,-16.5));
#35664=CARTESIAN_POINT('Origin',(0.,105.3,-16.5));
#35665=CARTESIAN_POINT('Origin',(0.,105.3,-16.5));
#35666=CARTESIAN_POINT('',(-11.,105.3,-16.5));
#35667=CARTESIAN_POINT('Origin',(0.,105.3,-16.5));
#35668=CARTESIAN_POINT('Origin',(0.,105.7,-16.5));
#35669=CARTESIAN_POINT('',(-7.2,93.7,-16.5));
#35670=CARTESIAN_POINT('',(-7.2,105.7,-16.5));
#35671=CARTESIAN_POINT('Origin',(0.,93.7,-16.5));
#35672=CARTESIAN_POINT('Origin',(-24.8,84.25,-24.75));
#35673=CARTESIAN_POINT('',(-24.55,84.5,0.));
#35674=CARTESIAN_POINT('',(-25.05,84.,0.));
#35675=CARTESIAN_POINT('',(-24.55,84.5,0.));
#35676=CARTESIAN_POINT('',(-25.05,84.,-33.));
#35677=CARTESIAN_POINT('',(-25.05,84.,-24.75));
#35678=CARTESIAN_POINT('',(-24.55,84.5,-33.));
#35679=CARTESIAN_POINT('',(-25.05,84.,-33.));
#35680=CARTESIAN_POINT('',(-24.55,84.5,-24.75));
#35681=CARTESIAN_POINT('Origin',(0.,84.25,0.));
#35682=CARTESIAN_POINT('',(24.55,84.5,3.00650789190675E-15));
#35683=CARTESIAN_POINT('',(25.05,84.,3.06774023186412E-15));
#35684=CARTESIAN_POINT('',(24.55,84.5,3.00650789190675E-15));
#35685=CARTESIAN_POINT('Origin',(0.,84.,0.));
#35686=CARTESIAN_POINT('Origin',(0.,84.5,0.));
#35687=CARTESIAN_POINT('Origin',(24.8,84.25,-8.25));
#35688=CARTESIAN_POINT('',(24.55,84.5,-33.));
#35689=CARTESIAN_POINT('',(25.05,84.,-33.));
#35690=CARTESIAN_POINT('',(24.55,84.5,-33.));
#35691=CARTESIAN_POINT('',(25.05,84.,-8.25));
#35692=CARTESIAN_POINT('',(24.55,84.5,-8.25));
#35693=CARTESIAN_POINT('Origin',(0.,84.25,-33.));
#35694=CARTESIAN_POINT('Origin',(0.,84.,-33.));
#35695=CARTESIAN_POINT('Origin',(0.,84.5,-33.));
#35696=CARTESIAN_POINT('Origin',(0.,84.,0.));
#35697=CARTESIAN_POINT('',(-24.55,86.05,0.));
#35698=CARTESIAN_POINT('',(-24.55,84.,0.));
#35699=CARTESIAN_POINT('',(24.55,86.05,3.00650789190675E-15));
#35700=CARTESIAN_POINT('Origin',(0.,86.05,0.));
#35701=CARTESIAN_POINT('',(24.55,84.,3.00650789190675E-15));
#35702=CARTESIAN_POINT('Origin',(-24.55,84.,-33.));
#35703=CARTESIAN_POINT('',(-24.55,86.05,-33.));
#35704=CARTESIAN_POINT('',(-24.55,84.,-33.));
#35705=CARTESIAN_POINT('',(-24.55,86.05,-33.));
#35706=CARTESIAN_POINT('Origin',(0.,84.,-16.5));
#35707=CARTESIAN_POINT('',(-30.5,84.,-67.5));
#35708=CARTESIAN_POINT('',(-40.,84.,-58.));
#35709=CARTESIAN_POINT('Origin',(-30.5,84.,-58.));
#35710=CARTESIAN_POINT('',(30.5,84.,-67.5));
#35711=CARTESIAN_POINT('',(15.25,84.,-67.5));
#35712=CARTESIAN_POINT('',(40.,84.,-58.));
#35713=CARTESIAN_POINT('Origin',(30.5,84.,-58.));
#35714=CARTESIAN_POINT('',(40.,84.,25.));
#35715=CARTESIAN_POINT('',(40.,84.,4.25));
#35716=CARTESIAN_POINT('',(30.5,84.,34.5));
#35717=CARTESIAN_POINT('Origin',(30.5,84.,25.));
#35718=CARTESIAN_POINT('',(-30.5,84.,34.5));
#35719=CARTESIAN_POINT('',(-15.25,84.,34.5));
#35720=CARTESIAN_POINT('',(-40.,84.,25.));
#35721=CARTESIAN_POINT('Origin',(-30.5,84.,25.));
#35722=CARTESIAN_POINT('',(-40.,84.,-37.25));
#35723=CARTESIAN_POINT('',(-35.8,84.,-55.));
#35724=CARTESIAN_POINT('Origin',(-30.5,84.,-55.));
#35725=CARTESIAN_POINT('',(25.2,84.,22.));
#35726=CARTESIAN_POINT('Origin',(30.5,84.,22.));
#35727=CARTESIAN_POINT('',(-35.8,84.,22.));
#35728=CARTESIAN_POINT('Origin',(-30.5,84.,22.));
#35729=CARTESIAN_POINT('',(25.2,84.,-55.));
#35730=CARTESIAN_POINT('Origin',(30.5,84.,-55.));
#35731=CARTESIAN_POINT('',(-34.51,84.,-16.5));
#35732=CARTESIAN_POINT('Origin',(-30.5,84.,-16.5));
#35733=CARTESIAN_POINT('',(26.49,84.,-16.5));
#35734=CARTESIAN_POINT('Origin',(30.5,84.,-16.5));
#35735=CARTESIAN_POINT('Origin',(22.2,84.25,-24.75));
#35736=CARTESIAN_POINT('',(22.45,84.5,2.74933206408581E-15));
#35737=CARTESIAN_POINT('',(21.95,84.,4.44089209850063E-15));
#35738=CARTESIAN_POINT('',(22.45,84.5,2.74933206408581E-15));
#35739=CARTESIAN_POINT('',(21.95,84.,-33.));
#35740=CARTESIAN_POINT('',(21.95,84.,-24.75));
#35741=CARTESIAN_POINT('',(22.45,84.5,-33.));
#35742=CARTESIAN_POINT('',(21.95,84.,-33.));
#35743=CARTESIAN_POINT('',(22.45,84.5,-24.75));
#35744=CARTESIAN_POINT('Origin',(0.,84.25,0.));
#35745=CARTESIAN_POINT('',(-22.45,84.5,0.));
#35746=CARTESIAN_POINT('',(-21.95,84.,5.37619944825688E-15));
#35747=CARTESIAN_POINT('',(-22.45,84.5,0.));
#35748=CARTESIAN_POINT('Origin',(0.,84.,0.));
#35749=CARTESIAN_POINT('Origin',(0.,84.5,0.));
#35750=CARTESIAN_POINT('Origin',(-22.2,84.25,-8.25));
#35751=CARTESIAN_POINT('',(-22.45,84.5,-33.));
#35752=CARTESIAN_POINT('',(-21.95,84.,-33.));
#35753=CARTESIAN_POINT('',(-22.45,84.5,-33.));
#35754=CARTESIAN_POINT('',(-21.95,84.,-8.25));
#35755=CARTESIAN_POINT('',(-22.45,84.5,-8.25));
#35756=CARTESIAN_POINT('Origin',(0.,84.25,-33.));
#35757=CARTESIAN_POINT('Origin',(0.,84.,-33.));
#35758=CARTESIAN_POINT('Origin',(0.,84.5,-33.));
#35759=CARTESIAN_POINT('Origin',(0.,84.,0.));
#35760=CARTESIAN_POINT('',(22.45,86.05,2.74933206408581E-15));
#35761=CARTESIAN_POINT('',(22.45,84.,2.74933206408581E-15));
#35762=CARTESIAN_POINT('',(-22.45,86.05,0.));
#35763=CARTESIAN_POINT('Origin',(0.,86.05,0.));
#35764=CARTESIAN_POINT('',(-22.45,84.,0.));
#35765=CARTESIAN_POINT('Origin',(22.45,84.,-33.));
#35766=CARTESIAN_POINT('',(22.45,86.05,-33.));
#35767=CARTESIAN_POINT('',(22.45,84.,-33.));
#35768=CARTESIAN_POINT('',(22.45,86.05,0.));
#35769=CARTESIAN_POINT('Origin',(0.,84.,-16.5));
#35770=CARTESIAN_POINT('Origin',(-30.5,105.45,22.));
#35771=CARTESIAN_POINT('',(-39.,105.7,19.0419601084502));
#35772=CARTESIAN_POINT('',(-39.25,105.45,22.));
#35773=CARTESIAN_POINT('Ctrl Pts',(-39.,105.7,19.0419601084503));
#35774=CARTESIAN_POINT('Ctrl Pts',(-39.25,105.45,20.5209800542251));
#35775=CARTESIAN_POINT('Ctrl Pts',(-39.25,105.45,22.));
#35776=CARTESIAN_POINT('',(-39.,105.2,22.));
#35777=CARTESIAN_POINT('',(-39.25,105.45,22.));
#35778=CARTESIAN_POINT('Origin',(-30.5,105.2,22.));
#35779=CARTESIAN_POINT('',(-39.,105.7,24.9580398915498));
#35780=CARTESIAN_POINT('Ctrl Pts',(-39.25,105.45,22.));
#35781=CARTESIAN_POINT('Ctrl Pts',(-39.25,105.45,23.4790199457749));
#35782=CARTESIAN_POINT('Ctrl Pts',(-39.,105.7,24.9580398915497));
#35783=CARTESIAN_POINT('Origin',(-30.5,105.7,22.));
#35784=CARTESIAN_POINT('Origin',(-39.75,104.95,-37.25));
#35785=CARTESIAN_POINT('',(-39.,105.7,-52.0419601084502));
#35786=CARTESIAN_POINT('',(-39.,105.7,-37.25));
#35787=CARTESIAN_POINT('',(-39.25,105.45,-55.));
#35788=CARTESIAN_POINT('Ctrl Pts',(-39.25,105.45,-55.));
#35789=CARTESIAN_POINT('Ctrl Pts',(-39.25,105.45,-53.5209800542251));
#35790=CARTESIAN_POINT('Ctrl Pts',(-39.,105.7,-52.0419601084503));
#35791=CARTESIAN_POINT('',(-39.,105.7,-57.9580398915498));
#35792=CARTESIAN_POINT('Ctrl Pts',(-39.,105.7,-57.9580398915497));
#35793=CARTESIAN_POINT('Ctrl Pts',(-39.25,105.45,-56.4790199457749));
#35794=CARTESIAN_POINT('Ctrl Pts',(-39.25,105.45,-55.));
#35795=CARTESIAN_POINT('',(-39.,105.7,-58.));
#35796=CARTESIAN_POINT('',(-39.,105.7,-37.25));
#35797=CARTESIAN_POINT('',(-40.1464466094067,104.553553390593,-58.));
#35798=CARTESIAN_POINT('',(-40.5,104.2,-58.));
#35799=CARTESIAN_POINT('',(-40.1464466094067,104.553553390593,25.));
#35800=CARTESIAN_POINT('',(-40.1464466094067,104.553553390593,-47.625));
#35801=CARTESIAN_POINT('',(-39.,105.7,25.));
#35802=CARTESIAN_POINT('',(-40.5,104.2,25.));
#35803=CARTESIAN_POINT('',(-39.,105.7,-37.25));
#35804=CARTESIAN_POINT('Origin',(-30.5,105.7,22.));
#35805=CARTESIAN_POINT('',(-39.,93.7,22.));
#35806=CARTESIAN_POINT('',(-39.,105.7,22.));
#35807=CARTESIAN_POINT('Origin',(-30.5,93.7,22.));
#35808=CARTESIAN_POINT('Origin',(-30.5,105.45,-55.));
#35809=CARTESIAN_POINT('',(-39.,105.2,-55.));
#35810=CARTESIAN_POINT('',(-39.25,105.45,-55.));
#35811=CARTESIAN_POINT('Origin',(-30.5,105.2,-55.));
#35812=CARTESIAN_POINT('Origin',(-30.5,105.7,-55.));
#35813=CARTESIAN_POINT('Origin',(-30.5,105.7,-55.));
#35814=CARTESIAN_POINT('',(-39.,93.7,-55.));
#35815=CARTESIAN_POINT('',(-39.,105.7,-55.));
#35816=CARTESIAN_POINT('Origin',(-30.5,93.7,-55.));
#35817=CARTESIAN_POINT('Origin',(30.5,105.45,-55.));
#35818=CARTESIAN_POINT('',(39.,105.7,-52.0419601084502));
#35819=CARTESIAN_POINT('',(39.25,105.45,-55.));
#35820=CARTESIAN_POINT('Ctrl Pts',(39.,105.7,-52.0419601084503));
#35821=CARTESIAN_POINT('Ctrl Pts',(39.25,105.45,-53.5209800542251));
#35822=CARTESIAN_POINT('Ctrl Pts',(39.25,105.45,-55.));
#35823=CARTESIAN_POINT('',(39.,105.2,-55.));
#35824=CARTESIAN_POINT('',(39.25,105.45,-55.));
#35825=CARTESIAN_POINT('',(22.,105.2,-55.));
#35826=CARTESIAN_POINT('Origin',(30.5,105.2,-55.));
#35827=CARTESIAN_POINT('Origin',(30.5,105.2,-55.));
#35828=CARTESIAN_POINT('',(39.,105.7,-57.9580398915498));
#35829=CARTESIAN_POINT('Ctrl Pts',(39.25,105.45,-55.));
#35830=CARTESIAN_POINT('Ctrl Pts',(39.25,105.45,-56.4790199457749));
#35831=CARTESIAN_POINT('Ctrl Pts',(39.,105.7,-57.9580398915497));
#35832=CARTESIAN_POINT('Origin',(30.5,105.7,-55.));
#35833=CARTESIAN_POINT('Origin',(39.75,104.95,4.25));
#35834=CARTESIAN_POINT('',(39.,105.7,19.0419601084502));
#35835=CARTESIAN_POINT('',(39.,105.7,4.25));
#35836=CARTESIAN_POINT('',(39.25,105.45,22.));
#35837=CARTESIAN_POINT('Ctrl Pts',(39.25,105.45,22.));
#35838=CARTESIAN_POINT('Ctrl Pts',(39.25,105.45,20.5209800542251));
#35839=CARTESIAN_POINT('Ctrl Pts',(39.,105.7,19.0419601084503));
#35840=CARTESIAN_POINT('',(39.,105.7,24.9580398915498));
#35841=CARTESIAN_POINT('Ctrl Pts',(39.,105.7,24.9580398915497));
#35842=CARTESIAN_POINT('Ctrl Pts',(39.25,105.45,23.4790199457749));
#35843=CARTESIAN_POINT('Ctrl Pts',(39.25,105.45,22.));
#35844=CARTESIAN_POINT('',(39.,105.7,25.));
#35845=CARTESIAN_POINT('',(39.,105.7,4.25));
#35846=CARTESIAN_POINT('',(40.1464466094067,104.553553390593,25.));
#35847=CARTESIAN_POINT('',(39.,105.7,25.));
#35848=CARTESIAN_POINT('',(40.1464466094067,104.553553390593,-58.));
#35849=CARTESIAN_POINT('',(40.1464466094067,104.553553390593,14.625));
#35850=CARTESIAN_POINT('',(39.,105.7,-58.));
#35851=CARTESIAN_POINT('',(40.5,104.2,-58.));
#35852=CARTESIAN_POINT('',(39.,105.7,4.25));
#35853=CARTESIAN_POINT('Origin',(30.5,105.7,-55.));
#35854=CARTESIAN_POINT('',(22.,93.7,-55.));
#35855=CARTESIAN_POINT('',(22.,105.7,-55.));
#35856=CARTESIAN_POINT('Origin',(30.5,93.7,-55.));
#35857=CARTESIAN_POINT('Origin',(30.5,105.45,22.));
#35858=CARTESIAN_POINT('',(39.,105.2,22.));
#35859=CARTESIAN_POINT('',(39.25,105.45,22.));
#35860=CARTESIAN_POINT('',(22.,105.2,22.));
#35861=CARTESIAN_POINT('Origin',(30.5,105.2,22.));
#35862=CARTESIAN_POINT('Origin',(30.5,105.2,22.));
#35863=CARTESIAN_POINT('Origin',(30.5,105.7,22.));
#35864=CARTESIAN_POINT('Origin',(30.5,105.7,22.));
#35865=CARTESIAN_POINT('',(22.,93.7,22.));
#35866=CARTESIAN_POINT('',(22.,105.7,22.));
#35867=CARTESIAN_POINT('Origin',(30.5,93.7,22.));
#35868=CARTESIAN_POINT('Origin',(-30.5,84.25,-58.));
#35869=CARTESIAN_POINT('',(-40.5,84.5,-58.));
#35870=CARTESIAN_POINT('',(-40.,84.,-58.));
#35871=CARTESIAN_POINT('',(-30.5,84.5,-68.));
#35872=CARTESIAN_POINT('Origin',(-30.5,84.5,-58.));
#35873=CARTESIAN_POINT('',(-30.5,84.5,-68.));
#35874=CARTESIAN_POINT('Origin',(-40.25,84.25,-37.25));
#35875=CARTESIAN_POINT('',(-40.5,84.5,25.));
#35876=CARTESIAN_POINT('',(-40.,84.,25.));
#35877=CARTESIAN_POINT('',(-40.5,84.5,-37.25));
#35878=CARTESIAN_POINT('Origin',(-30.5,84.25,25.));
#35879=CARTESIAN_POINT('',(-30.5,84.5,35.));
#35880=CARTESIAN_POINT('',(-30.5,84.,34.5));
#35881=CARTESIAN_POINT('Origin',(-30.5,84.5,25.));
#35882=CARTESIAN_POINT('Origin',(-15.25,84.25,34.75));
#35883=CARTESIAN_POINT('',(30.5,84.5,35.));
#35884=CARTESIAN_POINT('',(30.5,84.,34.5));
#35885=CARTESIAN_POINT('',(-15.25,84.5,35.));
#35886=CARTESIAN_POINT('Origin',(30.5,84.25,25.));
#35887=CARTESIAN_POINT('',(40.5,84.5,25.));
#35888=CARTESIAN_POINT('',(40.,84.,25.));
#35889=CARTESIAN_POINT('Origin',(30.5,84.5,25.));
#35890=CARTESIAN_POINT('Origin',(40.25,84.25,4.25));
#35891=CARTESIAN_POINT('',(40.5,84.5,-58.));
#35892=CARTESIAN_POINT('',(40.,84.,-58.));
#35893=CARTESIAN_POINT('',(40.5,84.5,4.25));
#35894=CARTESIAN_POINT('Origin',(30.5,84.25,-58.));
#35895=CARTESIAN_POINT('',(30.5,84.5,-68.));
#35896=CARTESIAN_POINT('',(30.5,84.,-67.5));
#35897=CARTESIAN_POINT('Origin',(30.5,84.5,-58.));
#35898=CARTESIAN_POINT('Origin',(15.25,84.25,-67.75));
#35899=CARTESIAN_POINT('',(15.25,84.5,-68.));
#35900=CARTESIAN_POINT('Origin',(40.5,84.,25.));
#35901=CARTESIAN_POINT('',(40.5,103.7,-58.));
#35902=CARTESIAN_POINT('',(40.5,84.,-58.));
#35903=CARTESIAN_POINT('',(40.5,103.7,25.));
#35904=CARTESIAN_POINT('',(40.5,103.7,14.625));
#35905=CARTESIAN_POINT('',(40.5,84.,25.));
#35906=CARTESIAN_POINT('Origin',(30.5,84.,-58.));
#35907=CARTESIAN_POINT('',(30.5,103.7,-68.));
#35908=CARTESIAN_POINT('',(30.5,84.,-68.));
#35909=CARTESIAN_POINT('Origin',(30.5,103.7,-58.));
#35910=CARTESIAN_POINT('Origin',(30.5,84.,-68.));
#35911=CARTESIAN_POINT('',(-30.5,103.7,-68.));
#35912=CARTESIAN_POINT('',(-30.5,84.,-68.));
#35913=CARTESIAN_POINT('',(22.875,103.7,-68.));
#35914=CARTESIAN_POINT('Origin',(-30.5,84.,-58.));
#35915=CARTESIAN_POINT('',(-40.5,103.7,-58.));
#35916=CARTESIAN_POINT('',(-40.5,84.,-58.));
#35917=CARTESIAN_POINT('Origin',(-30.5,103.7,-58.));
#35918=CARTESIAN_POINT('Origin',(40.3232233047034,104.126776695297,14.625));
#35919=CARTESIAN_POINT('',(40.5,103.7,-58.));
#35920=CARTESIAN_POINT('',(40.1464466094067,104.553553390593,25.));
#35921=CARTESIAN_POINT('Origin',(30.5,104.126776695297,-58.));
#35922=CARTESIAN_POINT('',(30.5,104.553553390593,-67.6464466094067));
#35923=CARTESIAN_POINT('',(30.5,103.7,-68.));
#35924=CARTESIAN_POINT('Origin',(30.5,104.553553390593,-58.));
#35925=CARTESIAN_POINT('Origin',(22.875,104.126776695297,-67.8232233047034));
#35926=CARTESIAN_POINT('',(-30.5,104.553553390593,-67.6464466094067));
#35927=CARTESIAN_POINT('',(-30.5,103.7,-68.));
#35928=CARTESIAN_POINT('',(22.875,104.553553390593,-67.6464466094067));
#35929=CARTESIAN_POINT('Origin',(-30.5,104.126776695297,-58.));
#35930=CARTESIAN_POINT('',(-40.5,103.7,-58.));
#35931=CARTESIAN_POINT('Origin',(-30.5,104.553553390593,-58.));
#35932=CARTESIAN_POINT('Origin',(-40.3232233047034,104.126776695297,-47.625));
#35933=CARTESIAN_POINT('',(-40.5,103.7,25.));
#35934=CARTESIAN_POINT('',(-40.5,103.7,25.));
#35935=CARTESIAN_POINT('',(-40.5,103.7,-47.625));
#35936=CARTESIAN_POINT('Origin',(-30.5,104.126776695297,25.));
#35937=CARTESIAN_POINT('',(-30.5,103.7,35.));
#35938=CARTESIAN_POINT('',(-30.5,104.553553390593,34.6464466094067));
#35939=CARTESIAN_POINT('',(-30.5,103.7,35.));
#35940=CARTESIAN_POINT('Origin',(-30.5,104.553553390593,25.));
#35941=CARTESIAN_POINT('Origin',(-30.5,103.7,25.));
#35942=CARTESIAN_POINT('Origin',(-22.875,104.126776695297,34.8232233047034));
#35943=CARTESIAN_POINT('',(30.5,103.7,35.));
#35944=CARTESIAN_POINT('',(30.5,104.553553390593,34.6464466094067));
#35945=CARTESIAN_POINT('',(30.5,103.7,35.));
#35946=CARTESIAN_POINT('',(-22.875,104.553553390593,34.6464466094067));
#35947=CARTESIAN_POINT('',(-22.875,103.7,35.));
#35948=CARTESIAN_POINT('Origin',(30.5,104.126776695297,25.));
#35949=CARTESIAN_POINT('Origin',(30.5,104.553553390593,25.));
#35950=CARTESIAN_POINT('Origin',(30.5,103.7,25.));
#35951=CARTESIAN_POINT('Origin',(-30.5,104.95,25.));
#35952=CARTESIAN_POINT('',(-30.5,105.7,33.5));
#35953=CARTESIAN_POINT('',(-30.5,104.2,35.));
#35954=CARTESIAN_POINT('Origin',(-30.5,105.7,25.));
#35955=CARTESIAN_POINT('Origin',(-15.25,104.95,34.25));
#35956=CARTESIAN_POINT('',(30.5,105.7,33.5));
#35957=CARTESIAN_POINT('',(30.5,104.2,35.));
#35958=CARTESIAN_POINT('',(-15.25,105.7,33.5));
#35959=CARTESIAN_POINT('Origin',(30.5,104.95,25.));
#35960=CARTESIAN_POINT('Origin',(30.5,105.7,25.));
#35961=CARTESIAN_POINT('Origin',(30.5,104.95,-58.));
#35962=CARTESIAN_POINT('',(30.5,105.7,-66.5));
#35963=CARTESIAN_POINT('',(30.5,104.2,-68.));
#35964=CARTESIAN_POINT('Origin',(30.5,105.7,-58.));
#35965=CARTESIAN_POINT('Origin',(15.25,104.95,-67.25));
#35966=CARTESIAN_POINT('',(-30.5,105.7,-66.5));
#35967=CARTESIAN_POINT('',(-30.5,104.2,-68.));
#35968=CARTESIAN_POINT('',(15.25,105.7,-66.5));
#35969=CARTESIAN_POINT('Origin',(-30.5,104.95,-58.));
#35970=CARTESIAN_POINT('Origin',(-30.5,105.7,-58.));
#35971=CARTESIAN_POINT('Origin',(0.,105.7,-16.5));
#35972=CARTESIAN_POINT('',(-11.,105.7,-16.5));
#35973=CARTESIAN_POINT('Origin',(0.,105.7,-16.5));
#35974=CARTESIAN_POINT('Origin',(0.,84.,-33.));
#35975=CARTESIAN_POINT('',(-22.45,86.05,-33.));
#35976=CARTESIAN_POINT('',(-22.45,84.,-33.));
#35977=CARTESIAN_POINT('Origin',(0.,86.05,-33.));
#35978=CARTESIAN_POINT('Origin',(-22.45,84.,0.));
#35979=CARTESIAN_POINT('',(-22.45,86.05,-33.));
#35980=CARTESIAN_POINT('Origin',(0.,84.,-33.));
#35981=CARTESIAN_POINT('',(24.55,86.05,-33.));
#35982=CARTESIAN_POINT('',(24.55,84.,-33.));
#35983=CARTESIAN_POINT('Origin',(0.,86.05,-33.));
#35984=CARTESIAN_POINT('Origin',(24.55,84.,0.));
#35985=CARTESIAN_POINT('',(24.55,86.05,0.));
#35986=CARTESIAN_POINT('Origin',(0.,86.05,-16.5));
#35987=CARTESIAN_POINT('Origin',(0.,105.7,-16.5));
#35988=CARTESIAN_POINT('',(-11.,105.7,-16.5));
#35989=CARTESIAN_POINT('Origin',(0.,93.7,-16.5));
#35990=CARTESIAN_POINT('Origin',(30.5,84.,-16.5));
#35991=CARTESIAN_POINT('',(26.49,92.1,-16.5));
#35992=CARTESIAN_POINT('',(26.49,84.,-16.5));
#35993=CARTESIAN_POINT('Origin',(30.5,92.1,-16.5));
#35994=CARTESIAN_POINT('Origin',(30.5,92.1,-16.5));
#35995=CARTESIAN_POINT('Origin',(-30.5,84.,-16.5));
#35996=CARTESIAN_POINT('',(-34.51,92.1,-16.5));
#35997=CARTESIAN_POINT('',(-34.51,84.,-16.5));
#35998=CARTESIAN_POINT('Origin',(-30.5,92.1,-16.5));
#35999=CARTESIAN_POINT('Origin',(-30.5,92.1,-16.5));
#36000=CARTESIAN_POINT('Origin',(30.5,93.7,-55.));
#36001=CARTESIAN_POINT('',(25.2,93.7,-55.));
#36002=CARTESIAN_POINT('Origin',(30.5,93.7,-55.));
#36003=CARTESIAN_POINT('',(25.2,93.7,-55.));
#36004=CARTESIAN_POINT('Origin',(-30.5,93.7,22.));
#36005=CARTESIAN_POINT('',(-35.8,93.7,22.));
#36006=CARTESIAN_POINT('Origin',(-30.5,93.7,22.));
#36007=CARTESIAN_POINT('',(-35.8,93.7,22.));
#36008=CARTESIAN_POINT('Origin',(30.5,93.7,22.));
#36009=CARTESIAN_POINT('',(25.2,93.7,22.));
#36010=CARTESIAN_POINT('Origin',(30.5,93.7,22.));
#36011=CARTESIAN_POINT('',(25.2,93.7,22.));
#36012=CARTESIAN_POINT('Origin',(-30.5,93.7,-55.));
#36013=CARTESIAN_POINT('',(-35.8,93.7,-55.));
#36014=CARTESIAN_POINT('Origin',(-30.5,93.7,-55.));
#36015=CARTESIAN_POINT('',(-35.8,93.7,-55.));
#36016=CARTESIAN_POINT('Origin',(30.5,93.7,-55.));
#36017=CARTESIAN_POINT('Origin',(-30.5,93.7,22.));
#36018=CARTESIAN_POINT('Origin',(30.5,93.7,22.));
#36019=CARTESIAN_POINT('Origin',(-30.5,93.7,-55.));
#36020=CARTESIAN_POINT('Origin',(30.5,84.,25.));
#36021=CARTESIAN_POINT('',(30.5,84.,35.));
#36022=CARTESIAN_POINT('Origin',(-30.5,84.,35.));
#36023=CARTESIAN_POINT('',(-30.5,84.,35.));
#36024=CARTESIAN_POINT('Origin',(-30.5,84.,25.));
#36025=CARTESIAN_POINT('',(-40.5,84.,25.));
#36026=CARTESIAN_POINT('Origin',(-40.5,84.,-58.));
#46367=UNCERTAINTY_MEASURE_WITH_UNIT(LENGTH_MEASURE(0.01),#46396,
'DISTANCE_ACCURACY_VALUE',
'Maximum model space distance between geometric entities at asserted c
onnectivities');
#46379=UNCERTAINTY_MEASURE_WITH_UNIT(LENGTH_MEASURE(0.01),#46396,
'DISTANCE_ACCURACY_VALUE',
'Maximum model space distance between geometric entities at asserted c
onnectivities');
#46383=(
GEOMETRIC_REPRESENTATION_CONTEXT(3)
GLOBAL_UNCERTAINTY_ASSIGNED_CONTEXT((#46367))
GLOBAL_UNIT_ASSIGNED_CONTEXT((#46396,#46398,#46399))
REPRESENTATION_CONTEXT('','3D')
);
#46395=(
GEOMETRIC_REPRESENTATION_CONTEXT(3)
GLOBAL_UNCERTAINTY_ASSIGNED_CONTEXT((#46379))
GLOBAL_UNIT_ASSIGNED_CONTEXT((#46396,#46398,#46399))
REPRESENTATION_CONTEXT('','3D')
);
#46396=(
LENGTH_UNIT()
NAMED_UNIT(*)
SI_UNIT(.MILLI.,.METRE.)
);
#46398=(
NAMED_UNIT(*)
PLANE_ANGLE_UNIT()
SI_UNIT($,.RADIAN.)
);
#46399=(
NAMED_UNIT(*)
SI_UNIT($,.STERADIAN.)
SOLID_ANGLE_UNIT()
);
#46403=SHAPE_DEFINITION_REPRESENTATION(#46418,#46458);
#46418=PRODUCT_DEFINITION_SHAPE('',$,#46474);
#46458=SHAPE_REPRESENTATION('',(#25562),#46383);
#46470=PRODUCT_DEFINITION_CONTEXT('part definition',#46517,'design');
#46474=PRODUCT_DEFINITION('2026-10-26-00-50-44-377','03_Rear_Cover',#46489,
#46470);
#46489=PRODUCT_DEFINITION_FORMATION('',$,#46522);
#46517=APPLICATION_CONTEXT(
'Core Data for Automotive Mechanical Design Process');
#46518=PRODUCT_CONTEXT('part definition',#46517,'mechanical');
#46522=PRODUCT('2026-10-26-00-50-44-377','03_Rear_Cover',$,(#46518));
#46604=COLOUR_RGB('Off White',0.89,0.88,0.83);
#46605=FILL_AREA_STYLE_COLOUR('',#46604);
#46606=FILL_AREA_STYLE('',(#46605));
#46607=SURFACE_STYLE_FILL_AREA(#46606);
#46608=SURFACE_SIDE_STYLE('',(#46607));
#46609=SURFACE_STYLE_USAGE(.BOTH.,#46608);
#46610=PRESENTATION_STYLE_ASSIGNMENT((#46609));
ENDSEC;
END-ISO-10303-21;
